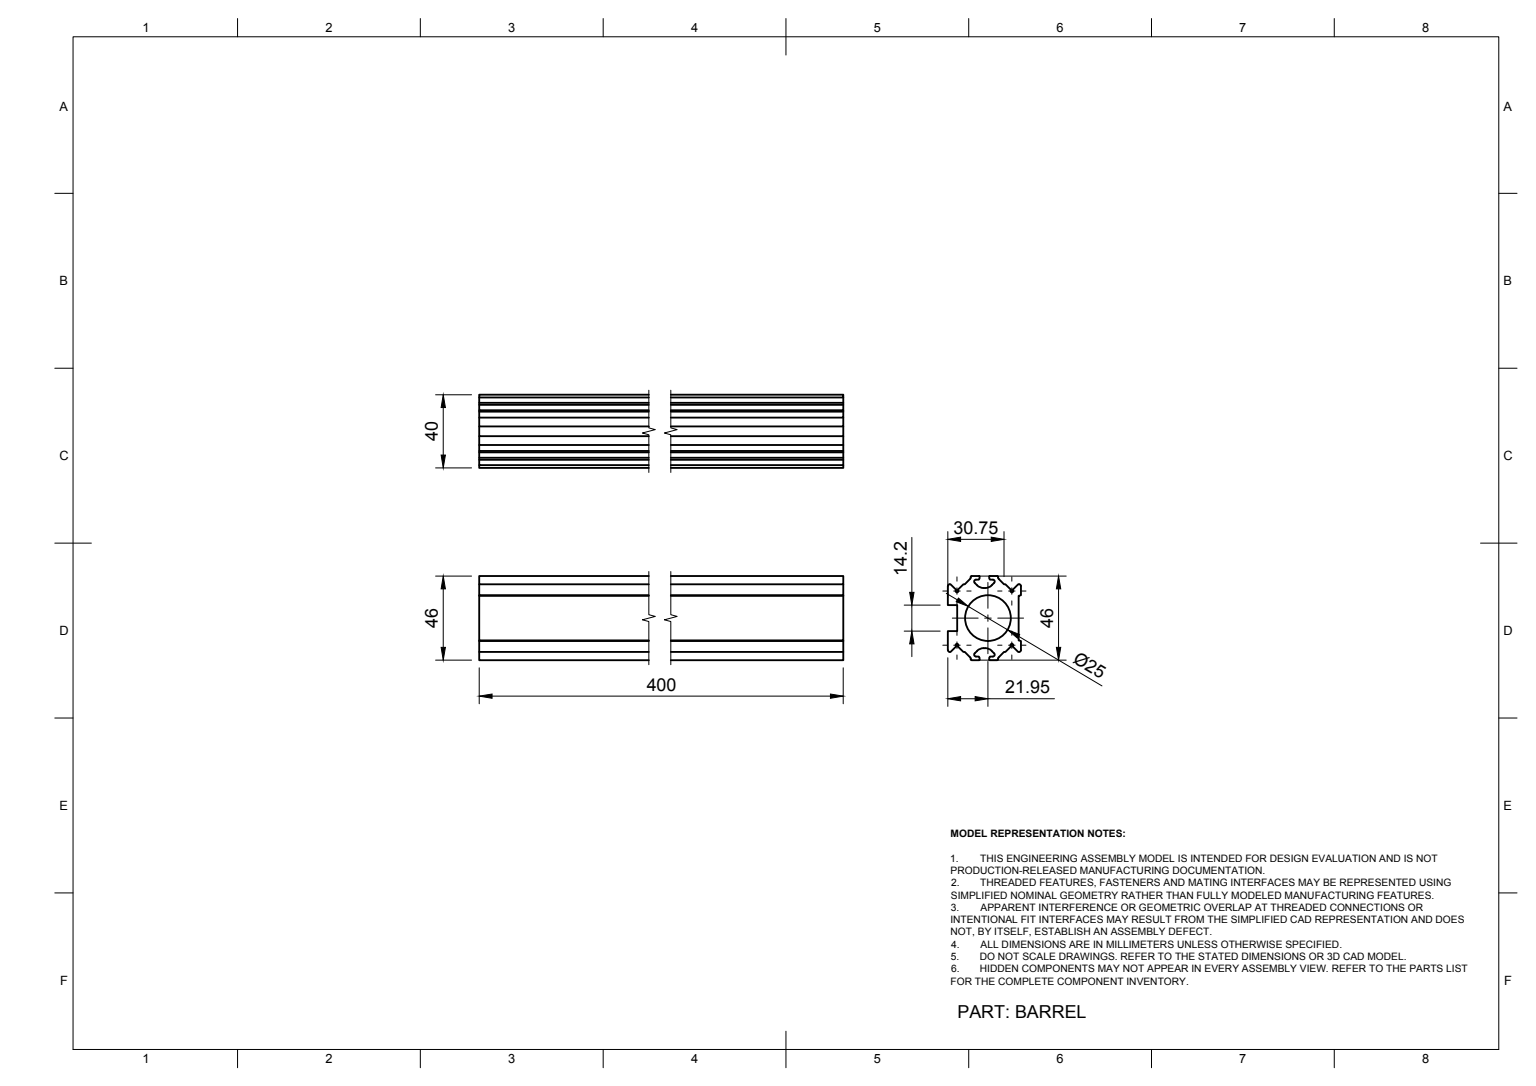
ISO-10303-21;
HEADER;
/* Generated by software containing ST-Developer
 * from STEP Tools, Inc. (www.steptools.com) 
 */

FILE_DESCRIPTION(
/* description */ (''),
/* implementation_level */ '2;1');

FILE_NAME(
/* name */ 'Barrel.step',
/* time_stamp */ '2026-10-05T11:01:41-07:00',
/* author */ (''),
/* organization */ (''),
/* preprocessor_version */ 'ST-DEVELOPER v20.2',
/* originating_system */ 'Autodesk Translation Framework v15.15.0.0',
/* authorisation */ '');

FILE_SCHEMA (('AUTOMOTIVE_DESIGN { 1 0 10303 214 3 1 1 }'));
ENDSEC;

DATA;
#10=MECHANICAL_DESIGN_GEOMETRIC_PRESENTATION_REPRESENTATION('',(#2144),#215609);
#218=FACE_BOUND('',#5274,.T.);
#219=FACE_BOUND('',#5276,.T.);
#2126=SHAPE_REPRESENTATION_RELATIONSHIP('SRR','None',#215651,#2135);
#2135=ADVANCED_BREP_SHAPE_REPRESENTATION('',(#2153),#215607);
#2144=STYLED_ITEM('',(#215698),#2153);
#2153=MANIFOLD_SOLID_BREP('Body1',#28087);
#2652=CYLINDRICAL_SURFACE('',#29551,12.5);
#2653=CYLINDRICAL_SURFACE('',#29554,0.999999999999998);
#2654=CYLINDRICAL_SURFACE('',#29562,1.);
#2655=CYLINDRICAL_SURFACE('',#29567,0.299999999999999);
#2656=CYLINDRICAL_SURFACE('',#29570,0.75);
#2657=CYLINDRICAL_SURFACE('',#29573,0.300000000000001);
#2658=CYLINDRICAL_SURFACE('',#29579,1.);
#2659=CYLINDRICAL_SURFACE('',#29583,0.499999999999999);
#2660=CYLINDRICAL_SURFACE('',#29587,0.299999999999998);
#2661=CYLINDRICAL_SURFACE('',#29593,0.999999999999998);
#2662=CYLINDRICAL_SURFACE('',#29597,5.);
#2663=CYLINDRICAL_SURFACE('',#29601,5.);
#2664=CYLINDRICAL_SURFACE('',#29605,0.999999999999996);
#2665=CYLINDRICAL_SURFACE('',#29611,0.299999999999998);
#2666=CYLINDRICAL_SURFACE('',#29615,0.5);
#2667=CYLINDRICAL_SURFACE('',#29619,1.);
#2668=CYLINDRICAL_SURFACE('',#29625,0.300000000000002);
#2669=CYLINDRICAL_SURFACE('',#29628,0.75000062202425);
#2670=CYLINDRICAL_SURFACE('',#29631,0.300000000000001);
#2671=CYLINDRICAL_SURFACE('',#29636,1.);
#2672=CYLINDRICAL_SURFACE('',#29644,1.);
#2673=CYLINDRICAL_SURFACE('',#29649,0.300000000000002);
#2674=CYLINDRICAL_SURFACE('',#29652,0.75);
#2675=CYLINDRICAL_SURFACE('',#29655,0.300000000000001);
#2676=CYLINDRICAL_SURFACE('',#29661,1.);
#2677=CYLINDRICAL_SURFACE('',#29665,0.500000000000003);
#2678=CYLINDRICAL_SURFACE('',#29669,0.299999999999998);
#2679=CYLINDRICAL_SURFACE('',#29675,1.);
#2680=CYLINDRICAL_SURFACE('',#29679,4.99999999999999);
#2681=CYLINDRICAL_SURFACE('',#29683,4.99999999999999);
#2682=CYLINDRICAL_SURFACE('',#29687,1.);
#2683=CYLINDRICAL_SURFACE('',#29693,0.300000000000003);
#2684=CYLINDRICAL_SURFACE('',#29697,0.5);
#2685=CYLINDRICAL_SURFACE('',#29701,1.);
#2686=CYLINDRICAL_SURFACE('',#29707,0.300000000000001);
#2687=CYLINDRICAL_SURFACE('',#29710,0.750000622024213);
#2688=CYLINDRICAL_SURFACE('',#29713,0.300000000000001);
#3822=FACE_OUTER_BOUND('',#5180,.T.);
#3823=FACE_OUTER_BOUND('',#5181,.T.);
#3824=FACE_OUTER_BOUND('',#5182,.T.);
#3825=FACE_OUTER_BOUND('',#5183,.T.);
#3826=FACE_OUTER_BOUND('',#5184,.T.);
#3827=FACE_OUTER_BOUND('',#5185,.T.);
#3828=FACE_OUTER_BOUND('',#5186,.T.);
#3829=FACE_OUTER_BOUND('',#5187,.T.);
#3830=FACE_OUTER_BOUND('',#5188,.T.);
#3831=FACE_OUTER_BOUND('',#5189,.T.);
#3832=FACE_OUTER_BOUND('',#5190,.T.);
#3833=FACE_OUTER_BOUND('',#5191,.T.);
#3834=FACE_OUTER_BOUND('',#5192,.T.);
#3835=FACE_OUTER_BOUND('',#5193,.T.);
#3836=FACE_OUTER_BOUND('',#5194,.T.);
#3837=FACE_OUTER_BOUND('',#5195,.T.);
#3838=FACE_OUTER_BOUND('',#5196,.T.);
#3839=FACE_OUTER_BOUND('',#5197,.T.);
#3840=FACE_OUTER_BOUND('',#5198,.T.);
#3841=FACE_OUTER_BOUND('',#5199,.T.);
#3842=FACE_OUTER_BOUND('',#5200,.T.);
#3843=FACE_OUTER_BOUND('',#5201,.T.);
#3844=FACE_OUTER_BOUND('',#5202,.T.);
#3845=FACE_OUTER_BOUND('',#5203,.T.);
#3846=FACE_OUTER_BOUND('',#5204,.T.);
#3847=FACE_OUTER_BOUND('',#5205,.T.);
#3848=FACE_OUTER_BOUND('',#5206,.T.);
#3849=FACE_OUTER_BOUND('',#5207,.T.);
#3850=FACE_OUTER_BOUND('',#5208,.T.);
#3851=FACE_OUTER_BOUND('',#5209,.T.);
#3852=FACE_OUTER_BOUND('',#5210,.T.);
#3853=FACE_OUTER_BOUND('',#5211,.T.);
#3854=FACE_OUTER_BOUND('',#5212,.T.);
#3855=FACE_OUTER_BOUND('',#5213,.T.);
#3856=FACE_OUTER_BOUND('',#5214,.T.);
#3857=FACE_OUTER_BOUND('',#5215,.T.);
#3858=FACE_OUTER_BOUND('',#5216,.T.);
#3859=FACE_OUTER_BOUND('',#5217,.T.);
#3860=FACE_OUTER_BOUND('',#5218,.T.);
#3861=FACE_OUTER_BOUND('',#5219,.T.);
#3862=FACE_OUTER_BOUND('',#5220,.T.);
#3863=FACE_OUTER_BOUND('',#5221,.T.);
#3864=FACE_OUTER_BOUND('',#5222,.T.);
#3865=FACE_OUTER_BOUND('',#5223,.T.);
#3866=FACE_OUTER_BOUND('',#5224,.T.);
#3867=FACE_OUTER_BOUND('',#5225,.T.);
#3868=FACE_OUTER_BOUND('',#5226,.T.);
#3869=FACE_OUTER_BOUND('',#5227,.T.);
#3870=FACE_OUTER_BOUND('',#5228,.T.);
#3871=FACE_OUTER_BOUND('',#5229,.T.);
#3872=FACE_OUTER_BOUND('',#5230,.T.);
#3873=FACE_OUTER_BOUND('',#5231,.T.);
#3874=FACE_OUTER_BOUND('',#5232,.T.);
#3875=FACE_OUTER_BOUND('',#5233,.T.);
#3876=FACE_OUTER_BOUND('',#5234,.T.);
#3877=FACE_OUTER_BOUND('',#5235,.T.);
#3878=FACE_OUTER_BOUND('',#5236,.T.);
#3879=FACE_OUTER_BOUND('',#5237,.T.);
#3880=FACE_OUTER_BOUND('',#5238,.T.);
#3881=FACE_OUTER_BOUND('',#5239,.T.);
#3882=FACE_OUTER_BOUND('',#5240,.T.);
#3883=FACE_OUTER_BOUND('',#5241,.T.);
#3884=FACE_OUTER_BOUND('',#5242,.T.);
#3885=FACE_OUTER_BOUND('',#5243,.T.);
#3886=FACE_OUTER_BOUND('',#5244,.T.);
#3887=FACE_OUTER_BOUND('',#5245,.T.);
#3888=FACE_OUTER_BOUND('',#5246,.T.);
#3889=FACE_OUTER_BOUND('',#5247,.T.);
#3890=FACE_OUTER_BOUND('',#5248,.T.);
#3891=FACE_OUTER_BOUND('',#5249,.T.);
#3892=FACE_OUTER_BOUND('',#5250,.T.);
#3893=FACE_OUTER_BOUND('',#5251,.T.);
#3894=FACE_OUTER_BOUND('',#5252,.T.);
#3895=FACE_OUTER_BOUND('',#5253,.T.);
#3896=FACE_OUTER_BOUND('',#5254,.T.);
#3897=FACE_OUTER_BOUND('',#5255,.T.);
#3898=FACE_OUTER_BOUND('',#5256,.T.);
#3899=FACE_OUTER_BOUND('',#5257,.T.);
#3900=FACE_OUTER_BOUND('',#5258,.T.);
#3901=FACE_OUTER_BOUND('',#5259,.T.);
#3902=FACE_OUTER_BOUND('',#5260,.T.);
#3903=FACE_OUTER_BOUND('',#5261,.T.);
#3904=FACE_OUTER_BOUND('',#5262,.T.);
#3905=FACE_OUTER_BOUND('',#5263,.T.);
#3906=FACE_OUTER_BOUND('',#5264,.T.);
#3907=FACE_OUTER_BOUND('',#5265,.T.);
#3908=FACE_OUTER_BOUND('',#5266,.T.);
#3909=FACE_OUTER_BOUND('',#5267,.T.);
#3910=FACE_OUTER_BOUND('',#5268,.T.);
#3911=FACE_OUTER_BOUND('',#5269,.T.);
#3912=FACE_OUTER_BOUND('',#5270,.T.);
#3913=FACE_OUTER_BOUND('',#5271,.T.);
#3914=FACE_OUTER_BOUND('',#5272,.T.);
#3915=FACE_OUTER_BOUND('',#5273,.T.);
#3916=FACE_OUTER_BOUND('',#5275,.T.);
#5180=EDGE_LOOP('',(#22991,#22992,#22993,#22994));
#5181=EDGE_LOOP('',(#22995,#22996,#22997,#22998));
#5182=EDGE_LOOP('',(#22999,#23000,#23001,#23002));
#5183=EDGE_LOOP('',(#23003,#23004,#23005,#23006));
#5184=EDGE_LOOP('',(#23007,#23008,#23009,#23010));
#5185=EDGE_LOOP('',(#23011,#23012,#23013,#23014));
#5186=EDGE_LOOP('',(#23015,#23016,#23017,#23018));
#5187=EDGE_LOOP('',(#23019,#23020,#23021,#23022));
#5188=EDGE_LOOP('',(#23023,#23024,#23025,#23026));
#5189=EDGE_LOOP('',(#23027,#23028,#23029,#23030));
#5190=EDGE_LOOP('',(#23031,#23032,#23033,#23034));
#5191=EDGE_LOOP('',(#23035,#23036,#23037,#23038));
#5192=EDGE_LOOP('',(#23039,#23040,#23041,#23042));
#5193=EDGE_LOOP('',(#23043,#23044,#23045,#23046));
#5194=EDGE_LOOP('',(#23047,#23048,#23049,#23050));
#5195=EDGE_LOOP('',(#23051,#23052,#23053,#23054));
#5196=EDGE_LOOP('',(#23055,#23056,#23057,#23058));
#5197=EDGE_LOOP('',(#23059,#23060,#23061,#23062));
#5198=EDGE_LOOP('',(#23063,#23064,#23065,#23066));
#5199=EDGE_LOOP('',(#23067,#23068,#23069,#23070));
#5200=EDGE_LOOP('',(#23071,#23072,#23073,#23074));
#5201=EDGE_LOOP('',(#23075,#23076,#23077,#23078));
#5202=EDGE_LOOP('',(#23079,#23080,#23081,#23082));
#5203=EDGE_LOOP('',(#23083,#23084,#23085,#23086));
#5204=EDGE_LOOP('',(#23087,#23088,#23089,#23090));
#5205=EDGE_LOOP('',(#23091,#23092,#23093,#23094));
#5206=EDGE_LOOP('',(#23095,#23096,#23097,#23098));
#5207=EDGE_LOOP('',(#23099,#23100,#23101,#23102));
#5208=EDGE_LOOP('',(#23103,#23104,#23105,#23106));
#5209=EDGE_LOOP('',(#23107,#23108,#23109,#23110));
#5210=EDGE_LOOP('',(#23111,#23112,#23113,#23114));
#5211=EDGE_LOOP('',(#23115,#23116,#23117,#23118));
#5212=EDGE_LOOP('',(#23119,#23120,#23121,#23122));
#5213=EDGE_LOOP('',(#23123,#23124,#23125,#23126));
#5214=EDGE_LOOP('',(#23127,#23128,#23129,#23130));
#5215=EDGE_LOOP('',(#23131,#23132,#23133,#23134));
#5216=EDGE_LOOP('',(#23135,#23136,#23137,#23138));
#5217=EDGE_LOOP('',(#23139,#23140,#23141,#23142));
#5218=EDGE_LOOP('',(#23143,#23144,#23145,#23146));
#5219=EDGE_LOOP('',(#23147,#23148,#23149,#23150));
#5220=EDGE_LOOP('',(#23151,#23152,#23153,#23154));
#5221=EDGE_LOOP('',(#23155,#23156,#23157,#23158));
#5222=EDGE_LOOP('',(#23159,#23160,#23161,#23162));
#5223=EDGE_LOOP('',(#23163,#23164,#23165,#23166));
#5224=EDGE_LOOP('',(#23167,#23168,#23169,#23170));
#5225=EDGE_LOOP('',(#23171,#23172,#23173,#23174));
#5226=EDGE_LOOP('',(#23175,#23176,#23177,#23178));
#5227=EDGE_LOOP('',(#23179,#23180,#23181,#23182));
#5228=EDGE_LOOP('',(#23183,#23184,#23185,#23186));
#5229=EDGE_LOOP('',(#23187,#23188,#23189,#23190));
#5230=EDGE_LOOP('',(#23191,#23192,#23193,#23194));
#5231=EDGE_LOOP('',(#23195,#23196,#23197,#23198));
#5232=EDGE_LOOP('',(#23199,#23200,#23201,#23202));
#5233=EDGE_LOOP('',(#23203,#23204,#23205,#23206));
#5234=EDGE_LOOP('',(#23207,#23208,#23209,#23210));
#5235=EDGE_LOOP('',(#23211,#23212,#23213,#23214));
#5236=EDGE_LOOP('',(#23215,#23216,#23217,#23218));
#5237=EDGE_LOOP('',(#23219,#23220,#23221,#23222));
#5238=EDGE_LOOP('',(#23223,#23224,#23225,#23226));
#5239=EDGE_LOOP('',(#23227,#23228,#23229,#23230));
#5240=EDGE_LOOP('',(#23231,#23232,#23233,#23234));
#5241=EDGE_LOOP('',(#23235,#23236,#23237,#23238));
#5242=EDGE_LOOP('',(#23239,#23240,#23241,#23242));
#5243=EDGE_LOOP('',(#23243,#23244,#23245,#23246));
#5244=EDGE_LOOP('',(#23247,#23248,#23249,#23250));
#5245=EDGE_LOOP('',(#23251,#23252,#23253,#23254));
#5246=EDGE_LOOP('',(#23255,#23256,#23257,#23258));
#5247=EDGE_LOOP('',(#23259,#23260,#23261,#23262));
#5248=EDGE_LOOP('',(#23263,#23264,#23265,#23266));
#5249=EDGE_LOOP('',(#23267,#23268,#23269,#23270));
#5250=EDGE_LOOP('',(#23271,#23272,#23273,#23274));
#5251=EDGE_LOOP('',(#23275,#23276,#23277,#23278));
#5252=EDGE_LOOP('',(#23279,#23280,#23281,#23282));
#5253=EDGE_LOOP('',(#23283,#23284,#23285,#23286));
#5254=EDGE_LOOP('',(#23287,#23288,#23289,#23290));
#5255=EDGE_LOOP('',(#23291,#23292,#23293,#23294));
#5256=EDGE_LOOP('',(#23295,#23296,#23297,#23298));
#5257=EDGE_LOOP('',(#23299,#23300,#23301,#23302));
#5258=EDGE_LOOP('',(#23303,#23304,#23305,#23306));
#5259=EDGE_LOOP('',(#23307,#23308,#23309,#23310));
#5260=EDGE_LOOP('',(#23311,#23312,#23313,#23314));
#5261=EDGE_LOOP('',(#23315,#23316,#23317,#23318));
#5262=EDGE_LOOP('',(#23319,#23320,#23321,#23322));
#5263=EDGE_LOOP('',(#23323,#23324,#23325,#23326));
#5264=EDGE_LOOP('',(#23327,#23328,#23329,#23330));
#5265=EDGE_LOOP('',(#23331,#23332,#23333,#23334));
#5266=EDGE_LOOP('',(#23335,#23336,#23337,#23338));
#5267=EDGE_LOOP('',(#23339,#23340,#23341,#23342));
#5268=EDGE_LOOP('',(#23343,#23344,#23345,#23346));
#5269=EDGE_LOOP('',(#23347,#23348,#23349,#23350));
#5270=EDGE_LOOP('',(#23351,#23352,#23353,#23354));
#5271=EDGE_LOOP('',(#23355,#23356,#23357,#23358));
#5272=EDGE_LOOP('',(#23359,#23360,#23361,#23362));
#5273=EDGE_LOOP('',(#23363,#23364,#23365,#23366,#23367,#23368,#23369,#23370,
#23371,#23372,#23373,#23374,#23375,#23376,#23377,#23378,#23379,#23380,#23381,
#23382,#23383,#23384,#23385,#23386,#23387,#23388,#23389,#23390,#23391,#23392,
#23393,#23394,#23395,#23396,#23397,#23398,#23399,#23400,#23401,#23402,#23403,
#23404,#23405,#23406,#23407,#23408,#23409,#23410,#23411,#23412,#23413,#23414,
#23415,#23416,#23417,#23418,#23419,#23420,#23421,#23422,#23423,#23424,#23425,
#23426,#23427,#23428,#23429,#23430,#23431,#23432,#23433,#23434,#23435,#23436,
#23437,#23438,#23439,#23440,#23441,#23442,#23443,#23444,#23445,#23446,#23447,
#23448,#23449,#23450,#23451,#23452,#23453,#23454));
#5274=EDGE_LOOP('',(#23455));
#5275=EDGE_LOOP('',(#23456,#23457,#23458,#23459,#23460,#23461,#23462,#23463,
#23464,#23465,#23466,#23467,#23468,#23469,#23470,#23471,#23472,#23473,#23474,
#23475,#23476,#23477,#23478,#23479,#23480,#23481,#23482,#23483,#23484,#23485,
#23486,#23487,#23488,#23489,#23490,#23491,#23492,#23493,#23494,#23495,#23496,
#23497,#23498,#23499,#23500,#23501,#23502,#23503,#23504,#23505,#23506,#23507,
#23508,#23509,#23510,#23511,#23512,#23513,#23514,#23515,#23516,#23517,#23518,
#23519,#23520,#23521,#23522,#23523,#23524,#23525,#23526,#23527,#23528,#23529,
#23530,#23531,#23532,#23533,#23534,#23535,#23536,#23537,#23538,#23539,#23540,
#23541,#23542,#23543,#23544,#23545,#23546,#23547));
#5276=EDGE_LOOP('',(#23548));
#6134=CIRCLE('',#29552,12.5);
#6135=CIRCLE('',#29553,12.5);
#6136=CIRCLE('',#29555,0.999999999999998);
#6137=CIRCLE('',#29556,0.999999999999998);
#6138=CIRCLE('',#29563,1.);
#6139=CIRCLE('',#29564,1.);
#6140=CIRCLE('',#29568,0.299999999999999);
#6141=CIRCLE('',#29569,0.299999999999999);
#6142=CIRCLE('',#29571,0.75);
#6143=CIRCLE('',#29572,0.75);
#6144=CIRCLE('',#29574,0.300000000000001);
#6145=CIRCLE('',#29575,0.300000000000001);
#6146=CIRCLE('',#29580,1.);
#6147=CIRCLE('',#29581,1.);
#6148=CIRCLE('',#29584,0.499999999999999);
#6149=CIRCLE('',#29585,0.499999999999999);
#6150=CIRCLE('',#29588,0.299999999999998);
#6151=CIRCLE('',#29589,0.299999999999998);
#6152=CIRCLE('',#29594,0.999999999999998);
#6153=CIRCLE('',#29595,0.999999999999998);
#6154=CIRCLE('',#29598,5.);
#6155=CIRCLE('',#29599,5.);
#6156=CIRCLE('',#29602,5.);
#6157=CIRCLE('',#29603,5.);
#6158=CIRCLE('',#29606,0.999999999999996);
#6159=CIRCLE('',#29607,0.999999999999996);
#6160=CIRCLE('',#29612,0.299999999999998);
#6161=CIRCLE('',#29613,0.299999999999998);
#6162=CIRCLE('',#29616,0.5);
#6163=CIRCLE('',#29617,0.5);
#6164=CIRCLE('',#29620,1.);
#6165=CIRCLE('',#29621,1.);
#6166=CIRCLE('',#29626,0.300000000000002);
#6167=CIRCLE('',#29627,0.300000000000002);
#6168=CIRCLE('',#29629,0.75000062202425);
#6169=CIRCLE('',#29630,0.75000062202425);
#6170=CIRCLE('',#29632,0.300000000000001);
#6171=CIRCLE('',#29633,0.300000000000001);
#6172=CIRCLE('',#29637,1.);
#6173=CIRCLE('',#29638,1.);
#6174=CIRCLE('',#29645,1.);
#6175=CIRCLE('',#29646,1.);
#6176=CIRCLE('',#29650,0.300000000000002);
#6177=CIRCLE('',#29651,0.300000000000002);
#6178=CIRCLE('',#29653,0.75);
#6179=CIRCLE('',#29654,0.75);
#6180=CIRCLE('',#29656,0.300000000000001);
#6181=CIRCLE('',#29657,0.300000000000001);
#6182=CIRCLE('',#29662,1.);
#6183=CIRCLE('',#29663,1.);
#6184=CIRCLE('',#29666,0.500000000000003);
#6185=CIRCLE('',#29667,0.500000000000003);
#6186=CIRCLE('',#29670,0.299999999999998);
#6187=CIRCLE('',#29671,0.299999999999998);
#6188=CIRCLE('',#29676,1.);
#6189=CIRCLE('',#29677,1.);
#6190=CIRCLE('',#29680,4.99999999999999);
#6191=CIRCLE('',#29681,4.99999999999999);
#6192=CIRCLE('',#29684,4.99999999999999);
#6193=CIRCLE('',#29685,4.99999999999999);
#6194=CIRCLE('',#29688,1.);
#6195=CIRCLE('',#29689,1.);
#6196=CIRCLE('',#29694,0.300000000000003);
#6197=CIRCLE('',#29695,0.300000000000003);
#6198=CIRCLE('',#29698,0.5);
#6199=CIRCLE('',#29699,0.5);
#6200=CIRCLE('',#29702,1.);
#6201=CIRCLE('',#29703,1.);
#6202=CIRCLE('',#29708,0.300000000000001);
#6203=CIRCLE('',#29709,0.300000000000001);
#6204=CIRCLE('',#29711,0.750000622024213);
#6205=CIRCLE('',#29712,0.750000622024213);
#6206=CIRCLE('',#29714,0.300000000000001);
#6207=CIRCLE('',#29715,0.300000000000001);
#7517=LINE('',#127846,#9362);
#7518=LINE('',#127853,#9363);
#7519=LINE('',#127856,#9364);
#7520=LINE('',#127859,#9365);
#7521=LINE('',#127861,#9366);
#7522=LINE('',#127862,#9367);
#7523=LINE('',#127865,#9368);
#7524=LINE('',#127867,#9369);
#7525=LINE('',#127868,#9370);
#7526=LINE('',#127871,#9371);
#7527=LINE('',#127873,#9372);
#7528=LINE('',#127874,#9373);
#7529=LINE('',#127877,#9374);
#7530=LINE('',#127879,#9375);
#7531=LINE('',#127880,#9376);
#7532=LINE('',#127883,#9377);
#7533=LINE('',#127885,#9378);
#7534=LINE('',#127886,#9379);
#7535=LINE('',#127892,#9380);
#7536=LINE('',#127895,#9381);
#7537=LINE('',#127897,#9382);
#7538=LINE('',#127898,#9383);
#7539=LINE('',#127901,#9384);
#7540=LINE('',#127903,#9385);
#7541=LINE('',#127904,#9386);
#7542=LINE('',#127910,#9387);
#7543=LINE('',#127916,#9388);
#7544=LINE('',#127922,#9389);
#7545=LINE('',#127925,#9390);
#7546=LINE('',#127927,#9391);
#7547=LINE('',#127928,#9392);
#7548=LINE('',#127931,#9393);
#7549=LINE('',#127933,#9394);
#7550=LINE('',#127934,#9395);
#7551=LINE('',#127937,#9396);
#7552=LINE('',#127939,#9397);
#7553=LINE('',#127940,#9398);
#7554=LINE('',#127946,#9399);
#7555=LINE('',#127949,#9400);
#7556=LINE('',#127951,#9401);
#7557=LINE('',#127952,#9402);
#7558=LINE('',#127958,#9403);
#7559=LINE('',#127961,#9404);
#7560=LINE('',#127963,#9405);
#7561=LINE('',#127964,#9406);
#7562=LINE('',#127970,#9407);
#7563=LINE('',#127973,#9408);
#7564=LINE('',#127975,#9409);
#7565=LINE('',#127976,#9410);
#7566=LINE('',#127979,#9411);
#7567=LINE('',#127981,#9412);
#7568=LINE('',#127982,#9413);
#7569=LINE('',#127985,#9414);
#7570=LINE('',#127987,#9415);
#7571=LINE('',#127988,#9416);
#7572=LINE('',#127994,#9417);
#7573=LINE('',#127997,#9418);
#7574=LINE('',#127999,#9419);
#7575=LINE('',#128000,#9420);
#7576=LINE('',#128006,#9421);
#7577=LINE('',#128009,#9422);
#7578=LINE('',#128011,#9423);
#7579=LINE('',#128012,#9424);
#7580=LINE('',#128018,#9425);
#7581=LINE('',#128021,#9426);
#7582=LINE('',#128023,#9427);
#7583=LINE('',#128024,#9428);
#7584=LINE('',#128030,#9429);
#7585=LINE('',#128033,#9430);
#7586=LINE('',#128035,#9431);
#7587=LINE('',#128036,#9432);
#7588=LINE('',#128039,#9433);
#7589=LINE('',#128041,#9434);
#7590=LINE('',#128042,#9435);
#7591=LINE('',#128045,#9436);
#7592=LINE('',#128047,#9437);
#7593=LINE('',#128048,#9438);
#7594=LINE('',#128054,#9439);
#7595=LINE('',#128057,#9440);
#7596=LINE('',#128059,#9441);
#7597=LINE('',#128060,#9442);
#7598=LINE('',#128066,#9443);
#7599=LINE('',#128069,#9444);
#7600=LINE('',#128071,#9445);
#7601=LINE('',#128072,#9446);
#7602=LINE('',#128078,#9447);
#7603=LINE('',#128081,#9448);
#7604=LINE('',#128083,#9449);
#7605=LINE('',#128084,#9450);
#7606=LINE('',#128087,#9451);
#7607=LINE('',#128089,#9452);
#7608=LINE('',#128090,#9453);
#7609=LINE('',#128093,#9454);
#7610=LINE('',#128095,#9455);
#7611=LINE('',#128096,#9456);
#7612=LINE('',#128102,#9457);
#7613=LINE('',#128108,#9458);
#7614=LINE('',#128114,#9459);
#7615=LINE('',#128117,#9460);
#7616=LINE('',#128119,#9461);
#7617=LINE('',#128120,#9462);
#7618=LINE('',#128123,#9463);
#7619=LINE('',#128125,#9464);
#7620=LINE('',#128126,#9465);
#7621=LINE('',#128132,#9466);
#7622=LINE('',#128135,#9467);
#7623=LINE('',#128137,#9468);
#7624=LINE('',#128138,#9469);
#7625=LINE('',#128141,#9470);
#7626=LINE('',#128143,#9471);
#7627=LINE('',#128144,#9472);
#7628=LINE('',#128147,#9473);
#7629=LINE('',#128149,#9474);
#7630=LINE('',#128150,#9475);
#7631=LINE('',#128153,#9476);
#7632=LINE('',#128155,#9477);
#7633=LINE('',#128156,#9478);
#7634=LINE('',#128159,#9479);
#7635=LINE('',#128161,#9480);
#7636=LINE('',#128162,#9481);
#7637=LINE('',#128168,#9482);
#7638=LINE('',#128171,#9483);
#7639=LINE('',#128173,#9484);
#7640=LINE('',#128174,#9485);
#7641=LINE('',#128177,#9486);
#7642=LINE('',#128179,#9487);
#7643=LINE('',#128180,#9488);
#7644=LINE('',#128186,#9489);
#7645=LINE('',#128192,#9490);
#7646=LINE('',#128198,#9491);
#7647=LINE('',#128201,#9492);
#7648=LINE('',#128203,#9493);
#7649=LINE('',#128204,#9494);
#7650=LINE('',#128207,#9495);
#7651=LINE('',#128209,#9496);
#7652=LINE('',#128210,#9497);
#7653=LINE('',#128213,#9498);
#7654=LINE('',#128215,#9499);
#7655=LINE('',#128216,#9500);
#7656=LINE('',#128222,#9501);
#7657=LINE('',#128225,#9502);
#7658=LINE('',#128227,#9503);
#7659=LINE('',#128228,#9504);
#7660=LINE('',#128234,#9505);
#7661=LINE('',#128237,#9506);
#7662=LINE('',#128239,#9507);
#7663=LINE('',#128240,#9508);
#7664=LINE('',#128246,#9509);
#7665=LINE('',#128249,#9510);
#7666=LINE('',#128251,#9511);
#7667=LINE('',#128252,#9512);
#7668=LINE('',#128255,#9513);
#7669=LINE('',#128257,#9514);
#7670=LINE('',#128258,#9515);
#7671=LINE('',#128261,#9516);
#7672=LINE('',#128263,#9517);
#7673=LINE('',#128264,#9518);
#7674=LINE('',#128270,#9519);
#7675=LINE('',#128273,#9520);
#7676=LINE('',#128275,#9521);
#7677=LINE('',#128276,#9522);
#7678=LINE('',#128282,#9523);
#7679=LINE('',#128285,#9524);
#7680=LINE('',#128287,#9525);
#7681=LINE('',#128288,#9526);
#7682=LINE('',#128294,#9527);
#7683=LINE('',#128297,#9528);
#7684=LINE('',#128299,#9529);
#7685=LINE('',#128300,#9530);
#7686=LINE('',#128306,#9531);
#7687=LINE('',#128309,#9532);
#7688=LINE('',#128311,#9533);
#7689=LINE('',#128312,#9534);
#7690=LINE('',#128315,#9535);
#7691=LINE('',#128317,#9536);
#7692=LINE('',#128318,#9537);
#7693=LINE('',#128321,#9538);
#7694=LINE('',#128323,#9539);
#7695=LINE('',#128324,#9540);
#7696=LINE('',#128330,#9541);
#7697=LINE('',#128333,#9542);
#7698=LINE('',#128335,#9543);
#7699=LINE('',#128336,#9544);
#7700=LINE('',#128342,#9545);
#7701=LINE('',#128345,#9546);
#7702=LINE('',#128347,#9547);
#7703=LINE('',#128348,#9548);
#7704=LINE('',#128354,#9549);
#7705=LINE('',#128357,#9550);
#7706=LINE('',#128359,#9551);
#7707=LINE('',#128360,#9552);
#7708=LINE('',#128363,#9553);
#7709=LINE('',#128365,#9554);
#7710=LINE('',#128366,#9555);
#7711=LINE('',#128369,#9556);
#7712=LINE('',#128371,#9557);
#7713=LINE('',#128372,#9558);
#7714=LINE('',#128378,#9559);
#7715=LINE('',#128384,#9560);
#7716=LINE('',#128390,#9561);
#7717=LINE('',#128393,#9562);
#7718=LINE('',#128395,#9563);
#7719=LINE('',#128396,#9564);
#7720=LINE('',#128398,#9565);
#7721=LINE('',#128399,#9566);
#9362=VECTOR('',#34135,12.5);
#9363=VECTOR('',#34142,10.);
#9364=VECTOR('',#34145,10.);
#9365=VECTOR('',#34148,10.);
#9366=VECTOR('',#34149,10.);
#9367=VECTOR('',#34150,10.);
#9368=VECTOR('',#34153,10.);
#9369=VECTOR('',#34154,10.);
#9370=VECTOR('',#34155,10.);
#9371=VECTOR('',#34158,10.);
#9372=VECTOR('',#34159,10.);
#9373=VECTOR('',#34160,10.);
#9374=VECTOR('',#34163,10.);
#9375=VECTOR('',#34164,10.);
#9376=VECTOR('',#34165,10.);
#9377=VECTOR('',#34168,10.);
#9378=VECTOR('',#34169,10.);
#9379=VECTOR('',#34170,10.);
#9380=VECTOR('',#34177,10.);
#9381=VECTOR('',#34180,10.);
#9382=VECTOR('',#34181,10.);
#9383=VECTOR('',#34182,10.);
#9384=VECTOR('',#34185,10.);
#9385=VECTOR('',#34186,10.);
#9386=VECTOR('',#34187,10.);
#9387=VECTOR('',#34194,10.);
#9388=VECTOR('',#34201,10.);
#9389=VECTOR('',#34208,10.);
#9390=VECTOR('',#34211,10.);
#9391=VECTOR('',#34212,10.);
#9392=VECTOR('',#34213,10.);
#9393=VECTOR('',#34216,10.);
#9394=VECTOR('',#34217,10.);
#9395=VECTOR('',#34218,10.);
#9396=VECTOR('',#34221,10.);
#9397=VECTOR('',#34222,10.);
#9398=VECTOR('',#34223,10.);
#9399=VECTOR('',#34230,10.);
#9400=VECTOR('',#34233,10.);
#9401=VECTOR('',#34234,10.);
#9402=VECTOR('',#34235,10.);
#9403=VECTOR('',#34242,10.);
#9404=VECTOR('',#34245,10.);
#9405=VECTOR('',#34246,10.);
#9406=VECTOR('',#34247,10.);
#9407=VECTOR('',#34254,10.);
#9408=VECTOR('',#34257,10.);
#9409=VECTOR('',#34258,10.);
#9410=VECTOR('',#34259,10.);
#9411=VECTOR('',#34262,10.);
#9412=VECTOR('',#34263,10.);
#9413=VECTOR('',#34264,10.);
#9414=VECTOR('',#34267,10.);
#9415=VECTOR('',#34268,10.);
#9416=VECTOR('',#34269,10.);
#9417=VECTOR('',#34276,10.);
#9418=VECTOR('',#34279,10.);
#9419=VECTOR('',#34280,10.);
#9420=VECTOR('',#34281,10.);
#9421=VECTOR('',#34288,10.);
#9422=VECTOR('',#34291,10.);
#9423=VECTOR('',#34292,10.);
#9424=VECTOR('',#34293,10.);
#9425=VECTOR('',#34300,10.);
#9426=VECTOR('',#34303,10.);
#9427=VECTOR('',#34304,10.);
#9428=VECTOR('',#34305,10.);
#9429=VECTOR('',#34312,10.);
#9430=VECTOR('',#34315,10.);
#9431=VECTOR('',#34316,10.);
#9432=VECTOR('',#34317,10.);
#9433=VECTOR('',#34320,10.);
#9434=VECTOR('',#34321,10.);
#9435=VECTOR('',#34322,10.);
#9436=VECTOR('',#34325,10.);
#9437=VECTOR('',#34326,10.);
#9438=VECTOR('',#34327,10.);
#9439=VECTOR('',#34334,10.);
#9440=VECTOR('',#34337,10.);
#9441=VECTOR('',#34338,10.);
#9442=VECTOR('',#34339,10.);
#9443=VECTOR('',#34346,10.);
#9444=VECTOR('',#34349,10.);
#9445=VECTOR('',#34350,10.);
#9446=VECTOR('',#34351,10.);
#9447=VECTOR('',#34358,10.);
#9448=VECTOR('',#34361,10.);
#9449=VECTOR('',#34362,10.);
#9450=VECTOR('',#34363,10.);
#9451=VECTOR('',#34366,10.);
#9452=VECTOR('',#34367,10.);
#9453=VECTOR('',#34368,10.);
#9454=VECTOR('',#34371,9.99999999999999);
#9455=VECTOR('',#34372,9.99999999999999);
#9456=VECTOR('',#34373,10.);
#9457=VECTOR('',#34380,10.);
#9458=VECTOR('',#34387,10.);
#9459=VECTOR('',#34394,10.);
#9460=VECTOR('',#34397,9.99999999999999);
#9461=VECTOR('',#34398,9.99999999999999);
#9462=VECTOR('',#34399,10.);
#9463=VECTOR('',#34402,10.);
#9464=VECTOR('',#34403,10.);
#9465=VECTOR('',#34404,10.);
#9466=VECTOR('',#34411,10.);
#9467=VECTOR('',#34414,10.);
#9468=VECTOR('',#34415,10.);
#9469=VECTOR('',#34416,10.);
#9470=VECTOR('',#34419,10.);
#9471=VECTOR('',#34420,10.);
#9472=VECTOR('',#34421,10.);
#9473=VECTOR('',#34424,10.);
#9474=VECTOR('',#34425,10.);
#9475=VECTOR('',#34426,10.);
#9476=VECTOR('',#34429,10.);
#9477=VECTOR('',#34430,10.);
#9478=VECTOR('',#34431,10.);
#9479=VECTOR('',#34434,10.);
#9480=VECTOR('',#34435,10.);
#9481=VECTOR('',#34436,10.);
#9482=VECTOR('',#34443,10.);
#9483=VECTOR('',#34446,10.);
#9484=VECTOR('',#34447,10.);
#9485=VECTOR('',#34448,10.);
#9486=VECTOR('',#34451,9.99999999999999);
#9487=VECTOR('',#34452,9.99999999999999);
#9488=VECTOR('',#34453,10.);
#9489=VECTOR('',#34460,10.);
#9490=VECTOR('',#34467,10.);
#9491=VECTOR('',#34474,10.);
#9492=VECTOR('',#34477,9.99999999999999);
#9493=VECTOR('',#34478,9.99999999999999);
#9494=VECTOR('',#34479,10.);
#9495=VECTOR('',#34482,10.);
#9496=VECTOR('',#34483,10.);
#9497=VECTOR('',#34484,10.);
#9498=VECTOR('',#34487,10.);
#9499=VECTOR('',#34488,10.);
#9500=VECTOR('',#34489,10.);
#9501=VECTOR('',#34496,10.);
#9502=VECTOR('',#34499,10.);
#9503=VECTOR('',#34500,10.);
#9504=VECTOR('',#34501,10.);
#9505=VECTOR('',#34508,10.);
#9506=VECTOR('',#34511,10.);
#9507=VECTOR('',#34512,10.);
#9508=VECTOR('',#34513,10.);
#9509=VECTOR('',#34520,10.);
#9510=VECTOR('',#34523,10.);
#9511=VECTOR('',#34524,10.);
#9512=VECTOR('',#34525,10.);
#9513=VECTOR('',#34528,10.);
#9514=VECTOR('',#34529,10.);
#9515=VECTOR('',#34530,10.);
#9516=VECTOR('',#34533,10.);
#9517=VECTOR('',#34534,10.);
#9518=VECTOR('',#34535,10.);
#9519=VECTOR('',#34542,10.);
#9520=VECTOR('',#34545,10.);
#9521=VECTOR('',#34546,10.);
#9522=VECTOR('',#34547,10.);
#9523=VECTOR('',#34554,10.);
#9524=VECTOR('',#34557,10.);
#9525=VECTOR('',#34558,10.);
#9526=VECTOR('',#34559,10.);
#9527=VECTOR('',#34566,10.);
#9528=VECTOR('',#34569,10.);
#9529=VECTOR('',#34570,10.);
#9530=VECTOR('',#34571,10.);
#9531=VECTOR('',#34578,10.);
#9532=VECTOR('',#34581,10.);
#9533=VECTOR('',#34582,10.);
#9534=VECTOR('',#34583,10.);
#9535=VECTOR('',#34586,10.);
#9536=VECTOR('',#34587,10.);
#9537=VECTOR('',#34588,10.);
#9538=VECTOR('',#34591,10.);
#9539=VECTOR('',#34592,10.);
#9540=VECTOR('',#34593,10.);
#9541=VECTOR('',#34600,10.);
#9542=VECTOR('',#34603,10.);
#9543=VECTOR('',#34604,10.);
#9544=VECTOR('',#34605,10.);
#9545=VECTOR('',#34612,10.);
#9546=VECTOR('',#34615,10.);
#9547=VECTOR('',#34616,10.);
#9548=VECTOR('',#34617,10.);
#9549=VECTOR('',#34624,10.);
#9550=VECTOR('',#34627,10.);
#9551=VECTOR('',#34628,10.);
#9552=VECTOR('',#34629,10.);
#9553=VECTOR('',#34632,10.);
#9554=VECTOR('',#34633,10.);
#9555=VECTOR('',#34634,10.);
#9556=VECTOR('',#34637,10.);
#9557=VECTOR('',#34638,10.);
#9558=VECTOR('',#34639,10.);
#9559=VECTOR('',#34646,10.);
#9560=VECTOR('',#34653,10.);
#9561=VECTOR('',#34660,10.);
#9562=VECTOR('',#34663,10.);
#9563=VECTOR('',#34664,10.);
#9564=VECTOR('',#34665,10.);
#9565=VECTOR('',#34668,10.);
#9566=VECTOR('',#34669,10.);
#11886=VERTEX_POINT('',#127843);
#11887=VERTEX_POINT('',#127845);
#11888=VERTEX_POINT('',#127849);
#11889=VERTEX_POINT('',#127850);
#11890=VERTEX_POINT('',#127852);
#11891=VERTEX_POINT('',#127854);
#11892=VERTEX_POINT('',#127858);
#11893=VERTEX_POINT('',#127860);
#11894=VERTEX_POINT('',#127864);
#11895=VERTEX_POINT('',#127866);
#11896=VERTEX_POINT('',#127870);
#11897=VERTEX_POINT('',#127872);
#11898=VERTEX_POINT('',#127876);
#11899=VERTEX_POINT('',#127878);
#11900=VERTEX_POINT('',#127882);
#11901=VERTEX_POINT('',#127884);
#11902=VERTEX_POINT('',#127888);
#11903=VERTEX_POINT('',#127890);
#11904=VERTEX_POINT('',#127894);
#11905=VERTEX_POINT('',#127896);
#11906=VERTEX_POINT('',#127900);
#11907=VERTEX_POINT('',#127902);
#11908=VERTEX_POINT('',#127906);
#11909=VERTEX_POINT('',#127908);
#11910=VERTEX_POINT('',#127912);
#11911=VERTEX_POINT('',#127914);
#11912=VERTEX_POINT('',#127918);
#11913=VERTEX_POINT('',#127920);
#11914=VERTEX_POINT('',#127924);
#11915=VERTEX_POINT('',#127926);
#11916=VERTEX_POINT('',#127930);
#11917=VERTEX_POINT('',#127932);
#11918=VERTEX_POINT('',#127936);
#11919=VERTEX_POINT('',#127938);
#11920=VERTEX_POINT('',#127942);
#11921=VERTEX_POINT('',#127944);
#11922=VERTEX_POINT('',#127948);
#11923=VERTEX_POINT('',#127950);
#11924=VERTEX_POINT('',#127954);
#11925=VERTEX_POINT('',#127956);
#11926=VERTEX_POINT('',#127960);
#11927=VERTEX_POINT('',#127962);
#11928=VERTEX_POINT('',#127966);
#11929=VERTEX_POINT('',#127968);
#11930=VERTEX_POINT('',#127972);
#11931=VERTEX_POINT('',#127974);
#11932=VERTEX_POINT('',#127978);
#11933=VERTEX_POINT('',#127980);
#11934=VERTEX_POINT('',#127984);
#11935=VERTEX_POINT('',#127986);
#11936=VERTEX_POINT('',#127990);
#11937=VERTEX_POINT('',#127992);
#11938=VERTEX_POINT('',#127996);
#11939=VERTEX_POINT('',#127998);
#11940=VERTEX_POINT('',#128002);
#11941=VERTEX_POINT('',#128004);
#11942=VERTEX_POINT('',#128008);
#11943=VERTEX_POINT('',#128010);
#11944=VERTEX_POINT('',#128014);
#11945=VERTEX_POINT('',#128016);
#11946=VERTEX_POINT('',#128020);
#11947=VERTEX_POINT('',#128022);
#11948=VERTEX_POINT('',#128026);
#11949=VERTEX_POINT('',#128028);
#11950=VERTEX_POINT('',#128032);
#11951=VERTEX_POINT('',#128034);
#11952=VERTEX_POINT('',#128038);
#11953=VERTEX_POINT('',#128040);
#11954=VERTEX_POINT('',#128044);
#11955=VERTEX_POINT('',#128046);
#11956=VERTEX_POINT('',#128050);
#11957=VERTEX_POINT('',#128052);
#11958=VERTEX_POINT('',#128056);
#11959=VERTEX_POINT('',#128058);
#11960=VERTEX_POINT('',#128062);
#11961=VERTEX_POINT('',#128064);
#11962=VERTEX_POINT('',#128068);
#11963=VERTEX_POINT('',#128070);
#11964=VERTEX_POINT('',#128074);
#11965=VERTEX_POINT('',#128076);
#11966=VERTEX_POINT('',#128080);
#11967=VERTEX_POINT('',#128082);
#11968=VERTEX_POINT('',#128086);
#11969=VERTEX_POINT('',#128088);
#11970=VERTEX_POINT('',#128092);
#11971=VERTEX_POINT('',#128094);
#11972=VERTEX_POINT('',#128098);
#11973=VERTEX_POINT('',#128100);
#11974=VERTEX_POINT('',#128104);
#11975=VERTEX_POINT('',#128106);
#11976=VERTEX_POINT('',#128110);
#11977=VERTEX_POINT('',#128112);
#11978=VERTEX_POINT('',#128116);
#11979=VERTEX_POINT('',#128118);
#11980=VERTEX_POINT('',#128122);
#11981=VERTEX_POINT('',#128124);
#11982=VERTEX_POINT('',#128128);
#11983=VERTEX_POINT('',#128130);
#11984=VERTEX_POINT('',#128134);
#11985=VERTEX_POINT('',#128136);
#11986=VERTEX_POINT('',#128140);
#11987=VERTEX_POINT('',#128142);
#11988=VERTEX_POINT('',#128146);
#11989=VERTEX_POINT('',#128148);
#11990=VERTEX_POINT('',#128152);
#11991=VERTEX_POINT('',#128154);
#11992=VERTEX_POINT('',#128158);
#11993=VERTEX_POINT('',#128160);
#11994=VERTEX_POINT('',#128164);
#11995=VERTEX_POINT('',#128166);
#11996=VERTEX_POINT('',#128170);
#11997=VERTEX_POINT('',#128172);
#11998=VERTEX_POINT('',#128176);
#11999=VERTEX_POINT('',#128178);
#12000=VERTEX_POINT('',#128182);
#12001=VERTEX_POINT('',#128184);
#12002=VERTEX_POINT('',#128188);
#12003=VERTEX_POINT('',#128190);
#12004=VERTEX_POINT('',#128194);
#12005=VERTEX_POINT('',#128196);
#12006=VERTEX_POINT('',#128200);
#12007=VERTEX_POINT('',#128202);
#12008=VERTEX_POINT('',#128206);
#12009=VERTEX_POINT('',#128208);
#12010=VERTEX_POINT('',#128212);
#12011=VERTEX_POINT('',#128214);
#12012=VERTEX_POINT('',#128218);
#12013=VERTEX_POINT('',#128220);
#12014=VERTEX_POINT('',#128224);
#12015=VERTEX_POINT('',#128226);
#12016=VERTEX_POINT('',#128230);
#12017=VERTEX_POINT('',#128232);
#12018=VERTEX_POINT('',#128236);
#12019=VERTEX_POINT('',#128238);
#12020=VERTEX_POINT('',#128242);
#12021=VERTEX_POINT('',#128244);
#12022=VERTEX_POINT('',#128248);
#12023=VERTEX_POINT('',#128250);
#12024=VERTEX_POINT('',#128254);
#12025=VERTEX_POINT('',#128256);
#12026=VERTEX_POINT('',#128260);
#12027=VERTEX_POINT('',#128262);
#12028=VERTEX_POINT('',#128266);
#12029=VERTEX_POINT('',#128268);
#12030=VERTEX_POINT('',#128272);
#12031=VERTEX_POINT('',#128274);
#12032=VERTEX_POINT('',#128278);
#12033=VERTEX_POINT('',#128280);
#12034=VERTEX_POINT('',#128284);
#12035=VERTEX_POINT('',#128286);
#12036=VERTEX_POINT('',#128290);
#12037=VERTEX_POINT('',#128292);
#12038=VERTEX_POINT('',#128296);
#12039=VERTEX_POINT('',#128298);
#12040=VERTEX_POINT('',#128302);
#12041=VERTEX_POINT('',#128304);
#12042=VERTEX_POINT('',#128308);
#12043=VERTEX_POINT('',#128310);
#12044=VERTEX_POINT('',#128314);
#12045=VERTEX_POINT('',#128316);
#12046=VERTEX_POINT('',#128320);
#12047=VERTEX_POINT('',#128322);
#12048=VERTEX_POINT('',#128326);
#12049=VERTEX_POINT('',#128328);
#12050=VERTEX_POINT('',#128332);
#12051=VERTEX_POINT('',#128334);
#12052=VERTEX_POINT('',#128338);
#12053=VERTEX_POINT('',#128340);
#12054=VERTEX_POINT('',#128344);
#12055=VERTEX_POINT('',#128346);
#12056=VERTEX_POINT('',#128350);
#12057=VERTEX_POINT('',#128352);
#12058=VERTEX_POINT('',#128356);
#12059=VERTEX_POINT('',#128358);
#12060=VERTEX_POINT('',#128362);
#12061=VERTEX_POINT('',#128364);
#12062=VERTEX_POINT('',#128368);
#12063=VERTEX_POINT('',#128370);
#12064=VERTEX_POINT('',#128374);
#12065=VERTEX_POINT('',#128376);
#12066=VERTEX_POINT('',#128380);
#12067=VERTEX_POINT('',#128382);
#12068=VERTEX_POINT('',#128386);
#12069=VERTEX_POINT('',#128388);
#12070=VERTEX_POINT('',#128392);
#12071=VERTEX_POINT('',#128394);
#15857=EDGE_CURVE('',#11886,#11886,#6134,.T.);
#15858=EDGE_CURVE('',#11886,#11887,#7517,.T.);
#15859=EDGE_CURVE('',#11887,#11887,#6135,.T.);
#15860=EDGE_CURVE('',#11888,#11889,#6136,.T.);
#15861=EDGE_CURVE('',#11889,#11890,#7518,.T.);
#15862=EDGE_CURVE('',#11891,#11890,#6137,.T.);
#15863=EDGE_CURVE('',#11888,#11891,#7519,.T.);
#15864=EDGE_CURVE('',#11888,#11892,#7520,.T.);
#15865=EDGE_CURVE('',#11893,#11891,#7521,.T.);
#15866=EDGE_CURVE('',#11892,#11893,#7522,.T.);
#15867=EDGE_CURVE('',#11894,#11892,#7523,.T.);
#15868=EDGE_CURVE('',#11895,#11893,#7524,.T.);
#15869=EDGE_CURVE('',#11894,#11895,#7525,.T.);
#15870=EDGE_CURVE('',#11896,#11894,#7526,.T.);
#15871=EDGE_CURVE('',#11897,#11895,#7527,.T.);
#15872=EDGE_CURVE('',#11896,#11897,#7528,.T.);
#15873=EDGE_CURVE('',#11896,#11898,#7529,.T.);
#15874=EDGE_CURVE('',#11899,#11897,#7530,.T.);
#15875=EDGE_CURVE('',#11898,#11899,#7531,.T.);
#15876=EDGE_CURVE('',#11900,#11898,#7532,.T.);
#15877=EDGE_CURVE('',#11901,#11899,#7533,.T.);
#15878=EDGE_CURVE('',#11900,#11901,#7534,.T.);
#15879=EDGE_CURVE('',#11902,#11900,#6138,.T.);
#15880=EDGE_CURVE('',#11903,#11901,#6139,.T.);
#15881=EDGE_CURVE('',#11902,#11903,#7535,.T.);
#15882=EDGE_CURVE('',#11902,#11904,#7536,.T.);
#15883=EDGE_CURVE('',#11905,#11903,#7537,.T.);
#15884=EDGE_CURVE('',#11904,#11905,#7538,.T.);
#15885=EDGE_CURVE('',#11904,#11906,#7539,.T.);
#15886=EDGE_CURVE('',#11907,#11905,#7540,.T.);
#15887=EDGE_CURVE('',#11906,#11907,#7541,.T.);
#15888=EDGE_CURVE('',#11908,#11906,#6140,.T.);
#15889=EDGE_CURVE('',#11909,#11907,#6141,.T.);
#15890=EDGE_CURVE('',#11908,#11909,#7542,.T.);
#15891=EDGE_CURVE('',#11908,#11910,#6142,.T.);
#15892=EDGE_CURVE('',#11911,#11909,#6143,.T.);
#15893=EDGE_CURVE('',#11910,#11911,#7543,.T.);
#15894=EDGE_CURVE('',#11912,#11910,#6144,.T.);
#15895=EDGE_CURVE('',#11913,#11911,#6145,.T.);
#15896=EDGE_CURVE('',#11912,#11913,#7544,.T.);
#15897=EDGE_CURVE('',#11914,#11912,#7545,.T.);
#15898=EDGE_CURVE('',#11915,#11913,#7546,.T.);
#15899=EDGE_CURVE('',#11914,#11915,#7547,.T.);
#15900=EDGE_CURVE('',#11914,#11916,#7548,.T.);
#15901=EDGE_CURVE('',#11917,#11915,#7549,.T.);
#15902=EDGE_CURVE('',#11916,#11917,#7550,.T.);
#15903=EDGE_CURVE('',#11916,#11918,#7551,.T.);
#15904=EDGE_CURVE('',#11919,#11917,#7552,.T.);
#15905=EDGE_CURVE('',#11918,#11919,#7553,.T.);
#15906=EDGE_CURVE('',#11918,#11920,#6146,.T.);
#15907=EDGE_CURVE('',#11921,#11919,#6147,.T.);
#15908=EDGE_CURVE('',#11920,#11921,#7554,.T.);
#15909=EDGE_CURVE('',#11920,#11922,#7555,.T.);
#15910=EDGE_CURVE('',#11923,#11921,#7556,.T.);
#15911=EDGE_CURVE('',#11922,#11923,#7557,.T.);
#15912=EDGE_CURVE('',#11924,#11922,#6148,.T.);
#15913=EDGE_CURVE('',#11925,#11923,#6149,.T.);
#15914=EDGE_CURVE('',#11924,#11925,#7558,.T.);
#15915=EDGE_CURVE('',#11924,#11926,#7559,.T.);
#15916=EDGE_CURVE('',#11927,#11925,#7560,.T.);
#15917=EDGE_CURVE('',#11926,#11927,#7561,.T.);
#15918=EDGE_CURVE('',#11928,#11926,#6150,.T.);
#15919=EDGE_CURVE('',#11929,#11927,#6151,.T.);
#15920=EDGE_CURVE('',#11928,#11929,#7562,.T.);
#15921=EDGE_CURVE('',#11928,#11930,#7563,.T.);
#15922=EDGE_CURVE('',#11931,#11929,#7564,.T.);
#15923=EDGE_CURVE('',#11930,#11931,#7565,.T.);
#15924=EDGE_CURVE('',#11930,#11932,#7566,.T.);
#15925=EDGE_CURVE('',#11933,#11931,#7567,.T.);
#15926=EDGE_CURVE('',#11932,#11933,#7568,.T.);
#15927=EDGE_CURVE('',#11932,#11934,#7569,.T.);
#15928=EDGE_CURVE('',#11935,#11933,#7570,.T.);
#15929=EDGE_CURVE('',#11934,#11935,#7571,.T.);
#15930=EDGE_CURVE('',#11934,#11936,#6152,.T.);
#15931=EDGE_CURVE('',#11937,#11935,#6153,.T.);
#15932=EDGE_CURVE('',#11936,#11937,#7572,.T.);
#15933=EDGE_CURVE('',#11936,#11938,#7573,.T.);
#15934=EDGE_CURVE('',#11939,#11937,#7574,.T.);
#15935=EDGE_CURVE('',#11938,#11939,#7575,.T.);
#15936=EDGE_CURVE('',#11938,#11940,#6154,.T.);
#15937=EDGE_CURVE('',#11941,#11939,#6155,.T.);
#15938=EDGE_CURVE('',#11940,#11941,#7576,.T.);
#15939=EDGE_CURVE('',#11942,#11940,#7577,.T.);
#15940=EDGE_CURVE('',#11943,#11941,#7578,.T.);
#15941=EDGE_CURVE('',#11942,#11943,#7579,.T.);
#15942=EDGE_CURVE('',#11942,#11944,#6156,.T.);
#15943=EDGE_CURVE('',#11945,#11943,#6157,.T.);
#15944=EDGE_CURVE('',#11944,#11945,#7580,.T.);
#15945=EDGE_CURVE('',#11946,#11944,#7581,.T.);
#15946=EDGE_CURVE('',#11947,#11945,#7582,.T.);
#15947=EDGE_CURVE('',#11946,#11947,#7583,.T.);
#15948=EDGE_CURVE('',#11946,#11948,#6158,.T.);
#15949=EDGE_CURVE('',#11949,#11947,#6159,.T.);
#15950=EDGE_CURVE('',#11948,#11949,#7584,.T.);
#15951=EDGE_CURVE('',#11950,#11948,#7585,.T.);
#15952=EDGE_CURVE('',#11951,#11949,#7586,.T.);
#15953=EDGE_CURVE('',#11950,#11951,#7587,.T.);
#15954=EDGE_CURVE('',#11952,#11950,#7588,.T.);
#15955=EDGE_CURVE('',#11953,#11951,#7589,.T.);
#15956=EDGE_CURVE('',#11952,#11953,#7590,.T.);
#15957=EDGE_CURVE('',#11954,#11952,#7591,.T.);
#15958=EDGE_CURVE('',#11955,#11953,#7592,.T.);
#15959=EDGE_CURVE('',#11954,#11955,#7593,.T.);
#15960=EDGE_CURVE('',#11956,#11954,#6160,.T.);
#15961=EDGE_CURVE('',#11957,#11955,#6161,.T.);
#15962=EDGE_CURVE('',#11956,#11957,#7594,.T.);
#15963=EDGE_CURVE('',#11958,#11956,#7595,.T.);
#15964=EDGE_CURVE('',#11959,#11957,#7596,.T.);
#15965=EDGE_CURVE('',#11958,#11959,#7597,.T.);
#15966=EDGE_CURVE('',#11960,#11958,#6162,.T.);
#15967=EDGE_CURVE('',#11961,#11959,#6163,.T.);
#15968=EDGE_CURVE('',#11960,#11961,#7598,.T.);
#15969=EDGE_CURVE('',#11962,#11960,#7599,.T.);
#15970=EDGE_CURVE('',#11963,#11961,#7600,.T.);
#15971=EDGE_CURVE('',#11962,#11963,#7601,.T.);
#15972=EDGE_CURVE('',#11962,#11964,#6164,.T.);
#15973=EDGE_CURVE('',#11965,#11963,#6165,.T.);
#15974=EDGE_CURVE('',#11964,#11965,#7602,.T.);
#15975=EDGE_CURVE('',#11966,#11964,#7603,.T.);
#15976=EDGE_CURVE('',#11967,#11965,#7604,.T.);
#15977=EDGE_CURVE('',#11966,#11967,#7605,.T.);
#15978=EDGE_CURVE('',#11968,#11966,#7606,.T.);
#15979=EDGE_CURVE('',#11969,#11967,#7607,.T.);
#15980=EDGE_CURVE('',#11968,#11969,#7608,.T.);
#15981=EDGE_CURVE('',#11968,#11970,#7609,.T.);
#15982=EDGE_CURVE('',#11971,#11969,#7610,.T.);
#15983=EDGE_CURVE('',#11970,#11971,#7611,.T.);
#15984=EDGE_CURVE('',#11972,#11970,#6166,.T.);
#15985=EDGE_CURVE('',#11973,#11971,#6167,.T.);
#15986=EDGE_CURVE('',#11972,#11973,#7612,.T.);
#15987=EDGE_CURVE('',#11972,#11974,#6168,.T.);
#15988=EDGE_CURVE('',#11975,#11973,#6169,.T.);
#15989=EDGE_CURVE('',#11974,#11975,#7613,.T.);
#15990=EDGE_CURVE('',#11976,#11974,#6170,.T.);
#15991=EDGE_CURVE('',#11977,#11975,#6171,.T.);
#15992=EDGE_CURVE('',#11976,#11977,#7614,.T.);
#15993=EDGE_CURVE('',#11978,#11976,#7615,.T.);
#15994=EDGE_CURVE('',#11979,#11977,#7616,.T.);
#15995=EDGE_CURVE('',#11978,#11979,#7617,.T.);
#15996=EDGE_CURVE('',#11980,#11978,#7618,.T.);
#15997=EDGE_CURVE('',#11981,#11979,#7619,.T.);
#15998=EDGE_CURVE('',#11980,#11981,#7620,.T.);
#15999=EDGE_CURVE('',#11982,#11980,#6172,.T.);
#16000=EDGE_CURVE('',#11983,#11981,#6173,.T.);
#16001=EDGE_CURVE('',#11982,#11983,#7621,.T.);
#16002=EDGE_CURVE('',#11984,#11982,#7622,.T.);
#16003=EDGE_CURVE('',#11985,#11983,#7623,.T.);
#16004=EDGE_CURVE('',#11984,#11985,#7624,.T.);
#16005=EDGE_CURVE('',#11986,#11984,#7625,.T.);
#16006=EDGE_CURVE('',#11987,#11985,#7626,.T.);
#16007=EDGE_CURVE('',#11986,#11987,#7627,.T.);
#16008=EDGE_CURVE('',#11986,#11988,#7628,.T.);
#16009=EDGE_CURVE('',#11989,#11987,#7629,.T.);
#16010=EDGE_CURVE('',#11988,#11989,#7630,.T.);
#16011=EDGE_CURVE('',#11988,#11990,#7631,.T.);
#16012=EDGE_CURVE('',#11991,#11989,#7632,.T.);
#16013=EDGE_CURVE('',#11990,#11991,#7633,.T.);
#16014=EDGE_CURVE('',#11990,#11992,#7634,.T.);
#16015=EDGE_CURVE('',#11993,#11991,#7635,.T.);
#16016=EDGE_CURVE('',#11992,#11993,#7636,.T.);
#16017=EDGE_CURVE('',#11994,#11992,#6174,.T.);
#16018=EDGE_CURVE('',#11995,#11993,#6175,.T.);
#16019=EDGE_CURVE('',#11994,#11995,#7637,.T.);
#16020=EDGE_CURVE('',#11994,#11996,#7638,.T.);
#16021=EDGE_CURVE('',#11997,#11995,#7639,.T.);
#16022=EDGE_CURVE('',#11996,#11997,#7640,.T.);
#16023=EDGE_CURVE('',#11996,#11998,#7641,.T.);
#16024=EDGE_CURVE('',#11999,#11997,#7642,.T.);
#16025=EDGE_CURVE('',#11998,#11999,#7643,.T.);
#16026=EDGE_CURVE('',#12000,#11998,#6176,.T.);
#16027=EDGE_CURVE('',#12001,#11999,#6177,.T.);
#16028=EDGE_CURVE('',#12000,#12001,#7644,.T.);
#16029=EDGE_CURVE('',#12000,#12002,#6178,.T.);
#16030=EDGE_CURVE('',#12003,#12001,#6179,.T.);
#16031=EDGE_CURVE('',#12002,#12003,#7645,.T.);
#16032=EDGE_CURVE('',#12004,#12002,#6180,.T.);
#16033=EDGE_CURVE('',#12005,#12003,#6181,.T.);
#16034=EDGE_CURVE('',#12004,#12005,#7646,.T.);
#16035=EDGE_CURVE('',#12006,#12004,#7647,.T.);
#16036=EDGE_CURVE('',#12007,#12005,#7648,.T.);
#16037=EDGE_CURVE('',#12006,#12007,#7649,.T.);
#16038=EDGE_CURVE('',#12006,#12008,#7650,.T.);
#16039=EDGE_CURVE('',#12009,#12007,#7651,.T.);
#16040=EDGE_CURVE('',#12008,#12009,#7652,.T.);
#16041=EDGE_CURVE('',#12008,#12010,#7653,.T.);
#16042=EDGE_CURVE('',#12011,#12009,#7654,.T.);
#16043=EDGE_CURVE('',#12010,#12011,#7655,.T.);
#16044=EDGE_CURVE('',#12010,#12012,#6182,.T.);
#16045=EDGE_CURVE('',#12013,#12011,#6183,.T.);
#16046=EDGE_CURVE('',#12012,#12013,#7656,.T.);
#16047=EDGE_CURVE('',#12012,#12014,#7657,.T.);
#16048=EDGE_CURVE('',#12015,#12013,#7658,.T.);
#16049=EDGE_CURVE('',#12014,#12015,#7659,.T.);
#16050=EDGE_CURVE('',#12016,#12014,#6184,.T.);
#16051=EDGE_CURVE('',#12017,#12015,#6185,.T.);
#16052=EDGE_CURVE('',#12016,#12017,#7660,.T.);
#16053=EDGE_CURVE('',#12016,#12018,#7661,.T.);
#16054=EDGE_CURVE('',#12019,#12017,#7662,.T.);
#16055=EDGE_CURVE('',#12018,#12019,#7663,.T.);
#16056=EDGE_CURVE('',#12020,#12018,#6186,.T.);
#16057=EDGE_CURVE('',#12021,#12019,#6187,.T.);
#16058=EDGE_CURVE('',#12020,#12021,#7664,.T.);
#16059=EDGE_CURVE('',#12020,#12022,#7665,.T.);
#16060=EDGE_CURVE('',#12023,#12021,#7666,.T.);
#16061=EDGE_CURVE('',#12022,#12023,#7667,.T.);
#16062=EDGE_CURVE('',#12022,#12024,#7668,.T.);
#16063=EDGE_CURVE('',#12025,#12023,#7669,.T.);
#16064=EDGE_CURVE('',#12024,#12025,#7670,.T.);
#16065=EDGE_CURVE('',#12024,#12026,#7671,.T.);
#16066=EDGE_CURVE('',#12027,#12025,#7672,.T.);
#16067=EDGE_CURVE('',#12026,#12027,#7673,.T.);
#16068=EDGE_CURVE('',#12026,#12028,#6188,.T.);
#16069=EDGE_CURVE('',#12029,#12027,#6189,.T.);
#16070=EDGE_CURVE('',#12028,#12029,#7674,.T.);
#16071=EDGE_CURVE('',#12028,#12030,#7675,.T.);
#16072=EDGE_CURVE('',#12031,#12029,#7676,.T.);
#16073=EDGE_CURVE('',#12030,#12031,#7677,.T.);
#16074=EDGE_CURVE('',#12030,#12032,#6190,.T.);
#16075=EDGE_CURVE('',#12033,#12031,#6191,.T.);
#16076=EDGE_CURVE('',#12032,#12033,#7678,.T.);
#16077=EDGE_CURVE('',#12032,#12034,#7679,.T.);
#16078=EDGE_CURVE('',#12035,#12033,#7680,.T.);
#16079=EDGE_CURVE('',#12034,#12035,#7681,.T.);
#16080=EDGE_CURVE('',#12034,#12036,#6192,.T.);
#16081=EDGE_CURVE('',#12037,#12035,#6193,.T.);
#16082=EDGE_CURVE('',#12036,#12037,#7682,.T.);
#16083=EDGE_CURVE('',#12038,#12036,#7683,.T.);
#16084=EDGE_CURVE('',#12039,#12037,#7684,.T.);
#16085=EDGE_CURVE('',#12038,#12039,#7685,.T.);
#16086=EDGE_CURVE('',#12038,#12040,#6194,.T.);
#16087=EDGE_CURVE('',#12041,#12039,#6195,.T.);
#16088=EDGE_CURVE('',#12040,#12041,#7686,.T.);
#16089=EDGE_CURVE('',#12042,#12040,#7687,.T.);
#16090=EDGE_CURVE('',#12043,#12041,#7688,.T.);
#16091=EDGE_CURVE('',#12042,#12043,#7689,.T.);
#16092=EDGE_CURVE('',#12044,#12042,#7690,.T.);
#16093=EDGE_CURVE('',#12045,#12043,#7691,.T.);
#16094=EDGE_CURVE('',#12044,#12045,#7692,.T.);
#16095=EDGE_CURVE('',#12046,#12044,#7693,.T.);
#16096=EDGE_CURVE('',#12047,#12045,#7694,.T.);
#16097=EDGE_CURVE('',#12046,#12047,#7695,.T.);
#16098=EDGE_CURVE('',#12048,#12046,#6196,.T.);
#16099=EDGE_CURVE('',#12049,#12047,#6197,.T.);
#16100=EDGE_CURVE('',#12048,#12049,#7696,.T.);
#16101=EDGE_CURVE('',#12050,#12048,#7697,.T.);
#16102=EDGE_CURVE('',#12051,#12049,#7698,.T.);
#16103=EDGE_CURVE('',#12050,#12051,#7699,.T.);
#16104=EDGE_CURVE('',#12052,#12050,#6198,.T.);
#16105=EDGE_CURVE('',#12053,#12051,#6199,.T.);
#16106=EDGE_CURVE('',#12052,#12053,#7700,.T.);
#16107=EDGE_CURVE('',#12054,#12052,#7701,.T.);
#16108=EDGE_CURVE('',#12055,#12053,#7702,.T.);
#16109=EDGE_CURVE('',#12054,#12055,#7703,.T.);
#16110=EDGE_CURVE('',#12054,#12056,#6200,.T.);
#16111=EDGE_CURVE('',#12057,#12055,#6201,.T.);
#16112=EDGE_CURVE('',#12056,#12057,#7704,.T.);
#16113=EDGE_CURVE('',#12058,#12056,#7705,.T.);
#16114=EDGE_CURVE('',#12059,#12057,#7706,.T.);
#16115=EDGE_CURVE('',#12058,#12059,#7707,.T.);
#16116=EDGE_CURVE('',#12060,#12058,#7708,.T.);
#16117=EDGE_CURVE('',#12061,#12059,#7709,.T.);
#16118=EDGE_CURVE('',#12060,#12061,#7710,.T.);
#16119=EDGE_CURVE('',#12060,#12062,#7711,.T.);
#16120=EDGE_CURVE('',#12063,#12061,#7712,.T.);
#16121=EDGE_CURVE('',#12062,#12063,#7713,.T.);
#16122=EDGE_CURVE('',#12064,#12062,#6202,.T.);
#16123=EDGE_CURVE('',#12065,#12063,#6203,.T.);
#16124=EDGE_CURVE('',#12064,#12065,#7714,.T.);
#16125=EDGE_CURVE('',#12064,#12066,#6204,.T.);
#16126=EDGE_CURVE('',#12067,#12065,#6205,.T.);
#16127=EDGE_CURVE('',#12066,#12067,#7715,.T.);
#16128=EDGE_CURVE('',#12068,#12066,#6206,.T.);
#16129=EDGE_CURVE('',#12069,#12067,#6207,.T.);
#16130=EDGE_CURVE('',#12068,#12069,#7716,.T.);
#16131=EDGE_CURVE('',#12070,#12068,#7717,.T.);
#16132=EDGE_CURVE('',#12071,#12069,#7718,.T.);
#16133=EDGE_CURVE('',#12070,#12071,#7719,.T.);
#16134=EDGE_CURVE('',#11889,#12070,#7720,.T.);
#16135=EDGE_CURVE('',#11890,#12071,#7721,.T.);
#22991=ORIENTED_EDGE('',*,*,#15857,.T.);
#22992=ORIENTED_EDGE('',*,*,#15858,.T.);
#22993=ORIENTED_EDGE('',*,*,#15859,.F.);
#22994=ORIENTED_EDGE('',*,*,#15858,.F.);
#22995=ORIENTED_EDGE('',*,*,#15860,.T.);
#22996=ORIENTED_EDGE('',*,*,#15861,.T.);
#22997=ORIENTED_EDGE('',*,*,#15862,.F.);
#22998=ORIENTED_EDGE('',*,*,#15863,.F.);
#22999=ORIENTED_EDGE('',*,*,#15864,.F.);
#23000=ORIENTED_EDGE('',*,*,#15863,.T.);
#23001=ORIENTED_EDGE('',*,*,#15865,.F.);
#23002=ORIENTED_EDGE('',*,*,#15866,.F.);
#23003=ORIENTED_EDGE('',*,*,#15867,.T.);
#23004=ORIENTED_EDGE('',*,*,#15866,.T.);
#23005=ORIENTED_EDGE('',*,*,#15868,.F.);
#23006=ORIENTED_EDGE('',*,*,#15869,.F.);
#23007=ORIENTED_EDGE('',*,*,#15870,.T.);
#23008=ORIENTED_EDGE('',*,*,#15869,.T.);
#23009=ORIENTED_EDGE('',*,*,#15871,.F.);
#23010=ORIENTED_EDGE('',*,*,#15872,.F.);
#23011=ORIENTED_EDGE('',*,*,#15873,.F.);
#23012=ORIENTED_EDGE('',*,*,#15872,.T.);
#23013=ORIENTED_EDGE('',*,*,#15874,.F.);
#23014=ORIENTED_EDGE('',*,*,#15875,.F.);
#23015=ORIENTED_EDGE('',*,*,#15876,.T.);
#23016=ORIENTED_EDGE('',*,*,#15875,.T.);
#23017=ORIENTED_EDGE('',*,*,#15877,.F.);
#23018=ORIENTED_EDGE('',*,*,#15878,.F.);
#23019=ORIENTED_EDGE('',*,*,#15879,.T.);
#23020=ORIENTED_EDGE('',*,*,#15878,.T.);
#23021=ORIENTED_EDGE('',*,*,#15880,.F.);
#23022=ORIENTED_EDGE('',*,*,#15881,.F.);
#23023=ORIENTED_EDGE('',*,*,#15882,.F.);
#23024=ORIENTED_EDGE('',*,*,#15881,.T.);
#23025=ORIENTED_EDGE('',*,*,#15883,.F.);
#23026=ORIENTED_EDGE('',*,*,#15884,.F.);
#23027=ORIENTED_EDGE('',*,*,#15885,.F.);
#23028=ORIENTED_EDGE('',*,*,#15884,.T.);
#23029=ORIENTED_EDGE('',*,*,#15886,.F.);
#23030=ORIENTED_EDGE('',*,*,#15887,.F.);
#23031=ORIENTED_EDGE('',*,*,#15888,.T.);
#23032=ORIENTED_EDGE('',*,*,#15887,.T.);
#23033=ORIENTED_EDGE('',*,*,#15889,.F.);
#23034=ORIENTED_EDGE('',*,*,#15890,.F.);
#23035=ORIENTED_EDGE('',*,*,#15891,.F.);
#23036=ORIENTED_EDGE('',*,*,#15890,.T.);
#23037=ORIENTED_EDGE('',*,*,#15892,.F.);
#23038=ORIENTED_EDGE('',*,*,#15893,.F.);
#23039=ORIENTED_EDGE('',*,*,#15894,.T.);
#23040=ORIENTED_EDGE('',*,*,#15893,.T.);
#23041=ORIENTED_EDGE('',*,*,#15895,.F.);
#23042=ORIENTED_EDGE('',*,*,#15896,.F.);
#23043=ORIENTED_EDGE('',*,*,#15897,.T.);
#23044=ORIENTED_EDGE('',*,*,#15896,.T.);
#23045=ORIENTED_EDGE('',*,*,#15898,.F.);
#23046=ORIENTED_EDGE('',*,*,#15899,.F.);
#23047=ORIENTED_EDGE('',*,*,#15900,.F.);
#23048=ORIENTED_EDGE('',*,*,#15899,.T.);
#23049=ORIENTED_EDGE('',*,*,#15901,.F.);
#23050=ORIENTED_EDGE('',*,*,#15902,.F.);
#23051=ORIENTED_EDGE('',*,*,#15903,.F.);
#23052=ORIENTED_EDGE('',*,*,#15902,.T.);
#23053=ORIENTED_EDGE('',*,*,#15904,.F.);
#23054=ORIENTED_EDGE('',*,*,#15905,.F.);
#23055=ORIENTED_EDGE('',*,*,#15906,.F.);
#23056=ORIENTED_EDGE('',*,*,#15905,.T.);
#23057=ORIENTED_EDGE('',*,*,#15907,.F.);
#23058=ORIENTED_EDGE('',*,*,#15908,.F.);
#23059=ORIENTED_EDGE('',*,*,#15909,.F.);
#23060=ORIENTED_EDGE('',*,*,#15908,.T.);
#23061=ORIENTED_EDGE('',*,*,#15910,.F.);
#23062=ORIENTED_EDGE('',*,*,#15911,.F.);
#23063=ORIENTED_EDGE('',*,*,#15912,.T.);
#23064=ORIENTED_EDGE('',*,*,#15911,.T.);
#23065=ORIENTED_EDGE('',*,*,#15913,.F.);
#23066=ORIENTED_EDGE('',*,*,#15914,.F.);
#23067=ORIENTED_EDGE('',*,*,#15915,.F.);
#23068=ORIENTED_EDGE('',*,*,#15914,.T.);
#23069=ORIENTED_EDGE('',*,*,#15916,.F.);
#23070=ORIENTED_EDGE('',*,*,#15917,.F.);
#23071=ORIENTED_EDGE('',*,*,#15918,.T.);
#23072=ORIENTED_EDGE('',*,*,#15917,.T.);
#23073=ORIENTED_EDGE('',*,*,#15919,.F.);
#23074=ORIENTED_EDGE('',*,*,#15920,.F.);
#23075=ORIENTED_EDGE('',*,*,#15921,.F.);
#23076=ORIENTED_EDGE('',*,*,#15920,.T.);
#23077=ORIENTED_EDGE('',*,*,#15922,.F.);
#23078=ORIENTED_EDGE('',*,*,#15923,.F.);
#23079=ORIENTED_EDGE('',*,*,#15924,.F.);
#23080=ORIENTED_EDGE('',*,*,#15923,.T.);
#23081=ORIENTED_EDGE('',*,*,#15925,.F.);
#23082=ORIENTED_EDGE('',*,*,#15926,.F.);
#23083=ORIENTED_EDGE('',*,*,#15927,.F.);
#23084=ORIENTED_EDGE('',*,*,#15926,.T.);
#23085=ORIENTED_EDGE('',*,*,#15928,.F.);
#23086=ORIENTED_EDGE('',*,*,#15929,.F.);
#23087=ORIENTED_EDGE('',*,*,#15930,.F.);
#23088=ORIENTED_EDGE('',*,*,#15929,.T.);
#23089=ORIENTED_EDGE('',*,*,#15931,.F.);
#23090=ORIENTED_EDGE('',*,*,#15932,.F.);
#23091=ORIENTED_EDGE('',*,*,#15933,.F.);
#23092=ORIENTED_EDGE('',*,*,#15932,.T.);
#23093=ORIENTED_EDGE('',*,*,#15934,.F.);
#23094=ORIENTED_EDGE('',*,*,#15935,.F.);
#23095=ORIENTED_EDGE('',*,*,#15936,.F.);
#23096=ORIENTED_EDGE('',*,*,#15935,.T.);
#23097=ORIENTED_EDGE('',*,*,#15937,.F.);
#23098=ORIENTED_EDGE('',*,*,#15938,.F.);
#23099=ORIENTED_EDGE('',*,*,#15939,.T.);
#23100=ORIENTED_EDGE('',*,*,#15938,.T.);
#23101=ORIENTED_EDGE('',*,*,#15940,.F.);
#23102=ORIENTED_EDGE('',*,*,#15941,.F.);
#23103=ORIENTED_EDGE('',*,*,#15942,.F.);
#23104=ORIENTED_EDGE('',*,*,#15941,.T.);
#23105=ORIENTED_EDGE('',*,*,#15943,.F.);
#23106=ORIENTED_EDGE('',*,*,#15944,.F.);
#23107=ORIENTED_EDGE('',*,*,#15945,.T.);
#23108=ORIENTED_EDGE('',*,*,#15944,.T.);
#23109=ORIENTED_EDGE('',*,*,#15946,.F.);
#23110=ORIENTED_EDGE('',*,*,#15947,.F.);
#23111=ORIENTED_EDGE('',*,*,#15948,.F.);
#23112=ORIENTED_EDGE('',*,*,#15947,.T.);
#23113=ORIENTED_EDGE('',*,*,#15949,.F.);
#23114=ORIENTED_EDGE('',*,*,#15950,.F.);
#23115=ORIENTED_EDGE('',*,*,#15951,.T.);
#23116=ORIENTED_EDGE('',*,*,#15950,.T.);
#23117=ORIENTED_EDGE('',*,*,#15952,.F.);
#23118=ORIENTED_EDGE('',*,*,#15953,.F.);
#23119=ORIENTED_EDGE('',*,*,#15954,.T.);
#23120=ORIENTED_EDGE('',*,*,#15953,.T.);
#23121=ORIENTED_EDGE('',*,*,#15955,.F.);
#23122=ORIENTED_EDGE('',*,*,#15956,.F.);
#23123=ORIENTED_EDGE('',*,*,#15957,.T.);
#23124=ORIENTED_EDGE('',*,*,#15956,.T.);
#23125=ORIENTED_EDGE('',*,*,#15958,.F.);
#23126=ORIENTED_EDGE('',*,*,#15959,.F.);
#23127=ORIENTED_EDGE('',*,*,#15960,.T.);
#23128=ORIENTED_EDGE('',*,*,#15959,.T.);
#23129=ORIENTED_EDGE('',*,*,#15961,.F.);
#23130=ORIENTED_EDGE('',*,*,#15962,.F.);
#23131=ORIENTED_EDGE('',*,*,#15963,.T.);
#23132=ORIENTED_EDGE('',*,*,#15962,.T.);
#23133=ORIENTED_EDGE('',*,*,#15964,.F.);
#23134=ORIENTED_EDGE('',*,*,#15965,.F.);
#23135=ORIENTED_EDGE('',*,*,#15966,.T.);
#23136=ORIENTED_EDGE('',*,*,#15965,.T.);
#23137=ORIENTED_EDGE('',*,*,#15967,.F.);
#23138=ORIENTED_EDGE('',*,*,#15968,.F.);
#23139=ORIENTED_EDGE('',*,*,#15969,.T.);
#23140=ORIENTED_EDGE('',*,*,#15968,.T.);
#23141=ORIENTED_EDGE('',*,*,#15970,.F.);
#23142=ORIENTED_EDGE('',*,*,#15971,.F.);
#23143=ORIENTED_EDGE('',*,*,#15972,.F.);
#23144=ORIENTED_EDGE('',*,*,#15971,.T.);
#23145=ORIENTED_EDGE('',*,*,#15973,.F.);
#23146=ORIENTED_EDGE('',*,*,#15974,.F.);
#23147=ORIENTED_EDGE('',*,*,#15975,.T.);
#23148=ORIENTED_EDGE('',*,*,#15974,.T.);
#23149=ORIENTED_EDGE('',*,*,#15976,.F.);
#23150=ORIENTED_EDGE('',*,*,#15977,.F.);
#23151=ORIENTED_EDGE('',*,*,#15978,.T.);
#23152=ORIENTED_EDGE('',*,*,#15977,.T.);
#23153=ORIENTED_EDGE('',*,*,#15979,.F.);
#23154=ORIENTED_EDGE('',*,*,#15980,.F.);
#23155=ORIENTED_EDGE('',*,*,#15981,.F.);
#23156=ORIENTED_EDGE('',*,*,#15980,.T.);
#23157=ORIENTED_EDGE('',*,*,#15982,.F.);
#23158=ORIENTED_EDGE('',*,*,#15983,.F.);
#23159=ORIENTED_EDGE('',*,*,#15984,.T.);
#23160=ORIENTED_EDGE('',*,*,#15983,.T.);
#23161=ORIENTED_EDGE('',*,*,#15985,.F.);
#23162=ORIENTED_EDGE('',*,*,#15986,.F.);
#23163=ORIENTED_EDGE('',*,*,#15987,.F.);
#23164=ORIENTED_EDGE('',*,*,#15986,.T.);
#23165=ORIENTED_EDGE('',*,*,#15988,.F.);
#23166=ORIENTED_EDGE('',*,*,#15989,.F.);
#23167=ORIENTED_EDGE('',*,*,#15990,.T.);
#23168=ORIENTED_EDGE('',*,*,#15989,.T.);
#23169=ORIENTED_EDGE('',*,*,#15991,.F.);
#23170=ORIENTED_EDGE('',*,*,#15992,.F.);
#23171=ORIENTED_EDGE('',*,*,#15993,.T.);
#23172=ORIENTED_EDGE('',*,*,#15992,.T.);
#23173=ORIENTED_EDGE('',*,*,#15994,.F.);
#23174=ORIENTED_EDGE('',*,*,#15995,.F.);
#23175=ORIENTED_EDGE('',*,*,#15996,.T.);
#23176=ORIENTED_EDGE('',*,*,#15995,.T.);
#23177=ORIENTED_EDGE('',*,*,#15997,.F.);
#23178=ORIENTED_EDGE('',*,*,#15998,.F.);
#23179=ORIENTED_EDGE('',*,*,#15999,.T.);
#23180=ORIENTED_EDGE('',*,*,#15998,.T.);
#23181=ORIENTED_EDGE('',*,*,#16000,.F.);
#23182=ORIENTED_EDGE('',*,*,#16001,.F.);
#23183=ORIENTED_EDGE('',*,*,#16002,.T.);
#23184=ORIENTED_EDGE('',*,*,#16001,.T.);
#23185=ORIENTED_EDGE('',*,*,#16003,.F.);
#23186=ORIENTED_EDGE('',*,*,#16004,.F.);
#23187=ORIENTED_EDGE('',*,*,#16005,.T.);
#23188=ORIENTED_EDGE('',*,*,#16004,.T.);
#23189=ORIENTED_EDGE('',*,*,#16006,.F.);
#23190=ORIENTED_EDGE('',*,*,#16007,.F.);
#23191=ORIENTED_EDGE('',*,*,#16008,.F.);
#23192=ORIENTED_EDGE('',*,*,#16007,.T.);
#23193=ORIENTED_EDGE('',*,*,#16009,.F.);
#23194=ORIENTED_EDGE('',*,*,#16010,.F.);
#23195=ORIENTED_EDGE('',*,*,#16011,.F.);
#23196=ORIENTED_EDGE('',*,*,#16010,.T.);
#23197=ORIENTED_EDGE('',*,*,#16012,.F.);
#23198=ORIENTED_EDGE('',*,*,#16013,.F.);
#23199=ORIENTED_EDGE('',*,*,#16014,.F.);
#23200=ORIENTED_EDGE('',*,*,#16013,.T.);
#23201=ORIENTED_EDGE('',*,*,#16015,.F.);
#23202=ORIENTED_EDGE('',*,*,#16016,.F.);
#23203=ORIENTED_EDGE('',*,*,#16017,.T.);
#23204=ORIENTED_EDGE('',*,*,#16016,.T.);
#23205=ORIENTED_EDGE('',*,*,#16018,.F.);
#23206=ORIENTED_EDGE('',*,*,#16019,.F.);
#23207=ORIENTED_EDGE('',*,*,#16020,.F.);
#23208=ORIENTED_EDGE('',*,*,#16019,.T.);
#23209=ORIENTED_EDGE('',*,*,#16021,.F.);
#23210=ORIENTED_EDGE('',*,*,#16022,.F.);
#23211=ORIENTED_EDGE('',*,*,#16023,.F.);
#23212=ORIENTED_EDGE('',*,*,#16022,.T.);
#23213=ORIENTED_EDGE('',*,*,#16024,.F.);
#23214=ORIENTED_EDGE('',*,*,#16025,.F.);
#23215=ORIENTED_EDGE('',*,*,#16026,.T.);
#23216=ORIENTED_EDGE('',*,*,#16025,.T.);
#23217=ORIENTED_EDGE('',*,*,#16027,.F.);
#23218=ORIENTED_EDGE('',*,*,#16028,.F.);
#23219=ORIENTED_EDGE('',*,*,#16029,.F.);
#23220=ORIENTED_EDGE('',*,*,#16028,.T.);
#23221=ORIENTED_EDGE('',*,*,#16030,.F.);
#23222=ORIENTED_EDGE('',*,*,#16031,.F.);
#23223=ORIENTED_EDGE('',*,*,#16032,.T.);
#23224=ORIENTED_EDGE('',*,*,#16031,.T.);
#23225=ORIENTED_EDGE('',*,*,#16033,.F.);
#23226=ORIENTED_EDGE('',*,*,#16034,.F.);
#23227=ORIENTED_EDGE('',*,*,#16035,.T.);
#23228=ORIENTED_EDGE('',*,*,#16034,.T.);
#23229=ORIENTED_EDGE('',*,*,#16036,.F.);
#23230=ORIENTED_EDGE('',*,*,#16037,.F.);
#23231=ORIENTED_EDGE('',*,*,#16038,.F.);
#23232=ORIENTED_EDGE('',*,*,#16037,.T.);
#23233=ORIENTED_EDGE('',*,*,#16039,.F.);
#23234=ORIENTED_EDGE('',*,*,#16040,.F.);
#23235=ORIENTED_EDGE('',*,*,#16041,.F.);
#23236=ORIENTED_EDGE('',*,*,#16040,.T.);
#23237=ORIENTED_EDGE('',*,*,#16042,.F.);
#23238=ORIENTED_EDGE('',*,*,#16043,.F.);
#23239=ORIENTED_EDGE('',*,*,#16044,.F.);
#23240=ORIENTED_EDGE('',*,*,#16043,.T.);
#23241=ORIENTED_EDGE('',*,*,#16045,.F.);
#23242=ORIENTED_EDGE('',*,*,#16046,.F.);
#23243=ORIENTED_EDGE('',*,*,#16047,.F.);
#23244=ORIENTED_EDGE('',*,*,#16046,.T.);
#23245=ORIENTED_EDGE('',*,*,#16048,.F.);
#23246=ORIENTED_EDGE('',*,*,#16049,.F.);
#23247=ORIENTED_EDGE('',*,*,#16050,.T.);
#23248=ORIENTED_EDGE('',*,*,#16049,.T.);
#23249=ORIENTED_EDGE('',*,*,#16051,.F.);
#23250=ORIENTED_EDGE('',*,*,#16052,.F.);
#23251=ORIENTED_EDGE('',*,*,#16053,.F.);
#23252=ORIENTED_EDGE('',*,*,#16052,.T.);
#23253=ORIENTED_EDGE('',*,*,#16054,.F.);
#23254=ORIENTED_EDGE('',*,*,#16055,.F.);
#23255=ORIENTED_EDGE('',*,*,#16056,.T.);
#23256=ORIENTED_EDGE('',*,*,#16055,.T.);
#23257=ORIENTED_EDGE('',*,*,#16057,.F.);
#23258=ORIENTED_EDGE('',*,*,#16058,.F.);
#23259=ORIENTED_EDGE('',*,*,#16059,.F.);
#23260=ORIENTED_EDGE('',*,*,#16058,.T.);
#23261=ORIENTED_EDGE('',*,*,#16060,.F.);
#23262=ORIENTED_EDGE('',*,*,#16061,.F.);
#23263=ORIENTED_EDGE('',*,*,#16062,.F.);
#23264=ORIENTED_EDGE('',*,*,#16061,.T.);
#23265=ORIENTED_EDGE('',*,*,#16063,.F.);
#23266=ORIENTED_EDGE('',*,*,#16064,.F.);
#23267=ORIENTED_EDGE('',*,*,#16065,.F.);
#23268=ORIENTED_EDGE('',*,*,#16064,.T.);
#23269=ORIENTED_EDGE('',*,*,#16066,.F.);
#23270=ORIENTED_EDGE('',*,*,#16067,.F.);
#23271=ORIENTED_EDGE('',*,*,#16068,.F.);
#23272=ORIENTED_EDGE('',*,*,#16067,.T.);
#23273=ORIENTED_EDGE('',*,*,#16069,.F.);
#23274=ORIENTED_EDGE('',*,*,#16070,.F.);
#23275=ORIENTED_EDGE('',*,*,#16071,.F.);
#23276=ORIENTED_EDGE('',*,*,#16070,.T.);
#23277=ORIENTED_EDGE('',*,*,#16072,.F.);
#23278=ORIENTED_EDGE('',*,*,#16073,.F.);
#23279=ORIENTED_EDGE('',*,*,#16074,.F.);
#23280=ORIENTED_EDGE('',*,*,#16073,.T.);
#23281=ORIENTED_EDGE('',*,*,#16075,.F.);
#23282=ORIENTED_EDGE('',*,*,#16076,.F.);
#23283=ORIENTED_EDGE('',*,*,#16077,.F.);
#23284=ORIENTED_EDGE('',*,*,#16076,.T.);
#23285=ORIENTED_EDGE('',*,*,#16078,.F.);
#23286=ORIENTED_EDGE('',*,*,#16079,.F.);
#23287=ORIENTED_EDGE('',*,*,#16080,.F.);
#23288=ORIENTED_EDGE('',*,*,#16079,.T.);
#23289=ORIENTED_EDGE('',*,*,#16081,.F.);
#23290=ORIENTED_EDGE('',*,*,#16082,.F.);
#23291=ORIENTED_EDGE('',*,*,#16083,.T.);
#23292=ORIENTED_EDGE('',*,*,#16082,.T.);
#23293=ORIENTED_EDGE('',*,*,#16084,.F.);
#23294=ORIENTED_EDGE('',*,*,#16085,.F.);
#23295=ORIENTED_EDGE('',*,*,#16086,.F.);
#23296=ORIENTED_EDGE('',*,*,#16085,.T.);
#23297=ORIENTED_EDGE('',*,*,#16087,.F.);
#23298=ORIENTED_EDGE('',*,*,#16088,.F.);
#23299=ORIENTED_EDGE('',*,*,#16089,.T.);
#23300=ORIENTED_EDGE('',*,*,#16088,.T.);
#23301=ORIENTED_EDGE('',*,*,#16090,.F.);
#23302=ORIENTED_EDGE('',*,*,#16091,.F.);
#23303=ORIENTED_EDGE('',*,*,#16092,.T.);
#23304=ORIENTED_EDGE('',*,*,#16091,.T.);
#23305=ORIENTED_EDGE('',*,*,#16093,.F.);
#23306=ORIENTED_EDGE('',*,*,#16094,.F.);
#23307=ORIENTED_EDGE('',*,*,#16095,.T.);
#23308=ORIENTED_EDGE('',*,*,#16094,.T.);
#23309=ORIENTED_EDGE('',*,*,#16096,.F.);
#23310=ORIENTED_EDGE('',*,*,#16097,.F.);
#23311=ORIENTED_EDGE('',*,*,#16098,.T.);
#23312=ORIENTED_EDGE('',*,*,#16097,.T.);
#23313=ORIENTED_EDGE('',*,*,#16099,.F.);
#23314=ORIENTED_EDGE('',*,*,#16100,.F.);
#23315=ORIENTED_EDGE('',*,*,#16101,.T.);
#23316=ORIENTED_EDGE('',*,*,#16100,.T.);
#23317=ORIENTED_EDGE('',*,*,#16102,.F.);
#23318=ORIENTED_EDGE('',*,*,#16103,.F.);
#23319=ORIENTED_EDGE('',*,*,#16104,.T.);
#23320=ORIENTED_EDGE('',*,*,#16103,.T.);
#23321=ORIENTED_EDGE('',*,*,#16105,.F.);
#23322=ORIENTED_EDGE('',*,*,#16106,.F.);
#23323=ORIENTED_EDGE('',*,*,#16107,.T.);
#23324=ORIENTED_EDGE('',*,*,#16106,.T.);
#23325=ORIENTED_EDGE('',*,*,#16108,.F.);
#23326=ORIENTED_EDGE('',*,*,#16109,.F.);
#23327=ORIENTED_EDGE('',*,*,#16110,.F.);
#23328=ORIENTED_EDGE('',*,*,#16109,.T.);
#23329=ORIENTED_EDGE('',*,*,#16111,.F.);
#23330=ORIENTED_EDGE('',*,*,#16112,.F.);
#23331=ORIENTED_EDGE('',*,*,#16113,.T.);
#23332=ORIENTED_EDGE('',*,*,#16112,.T.);
#23333=ORIENTED_EDGE('',*,*,#16114,.F.);
#23334=ORIENTED_EDGE('',*,*,#16115,.F.);
#23335=ORIENTED_EDGE('',*,*,#16116,.T.);
#23336=ORIENTED_EDGE('',*,*,#16115,.T.);
#23337=ORIENTED_EDGE('',*,*,#16117,.F.);
#23338=ORIENTED_EDGE('',*,*,#16118,.F.);
#23339=ORIENTED_EDGE('',*,*,#16119,.F.);
#23340=ORIENTED_EDGE('',*,*,#16118,.T.);
#23341=ORIENTED_EDGE('',*,*,#16120,.F.);
#23342=ORIENTED_EDGE('',*,*,#16121,.F.);
#23343=ORIENTED_EDGE('',*,*,#16122,.T.);
#23344=ORIENTED_EDGE('',*,*,#16121,.T.);
#23345=ORIENTED_EDGE('',*,*,#16123,.F.);
#23346=ORIENTED_EDGE('',*,*,#16124,.F.);
#23347=ORIENTED_EDGE('',*,*,#16125,.F.);
#23348=ORIENTED_EDGE('',*,*,#16124,.T.);
#23349=ORIENTED_EDGE('',*,*,#16126,.F.);
#23350=ORIENTED_EDGE('',*,*,#16127,.F.);
#23351=ORIENTED_EDGE('',*,*,#16128,.T.);
#23352=ORIENTED_EDGE('',*,*,#16127,.T.);
#23353=ORIENTED_EDGE('',*,*,#16129,.F.);
#23354=ORIENTED_EDGE('',*,*,#16130,.F.);
#23355=ORIENTED_EDGE('',*,*,#16131,.T.);
#23356=ORIENTED_EDGE('',*,*,#16130,.T.);
#23357=ORIENTED_EDGE('',*,*,#16132,.F.);
#23358=ORIENTED_EDGE('',*,*,#16133,.F.);
#23359=ORIENTED_EDGE('',*,*,#16134,.T.);
#23360=ORIENTED_EDGE('',*,*,#16133,.T.);
#23361=ORIENTED_EDGE('',*,*,#16135,.F.);
#23362=ORIENTED_EDGE('',*,*,#15861,.F.);
#23363=ORIENTED_EDGE('',*,*,#16135,.T.);
#23364=ORIENTED_EDGE('',*,*,#16132,.T.);
#23365=ORIENTED_EDGE('',*,*,#16129,.T.);
#23366=ORIENTED_EDGE('',*,*,#16126,.T.);
#23367=ORIENTED_EDGE('',*,*,#16123,.T.);
#23368=ORIENTED_EDGE('',*,*,#16120,.T.);
#23369=ORIENTED_EDGE('',*,*,#16117,.T.);
#23370=ORIENTED_EDGE('',*,*,#16114,.T.);
#23371=ORIENTED_EDGE('',*,*,#16111,.T.);
#23372=ORIENTED_EDGE('',*,*,#16108,.T.);
#23373=ORIENTED_EDGE('',*,*,#16105,.T.);
#23374=ORIENTED_EDGE('',*,*,#16102,.T.);
#23375=ORIENTED_EDGE('',*,*,#16099,.T.);
#23376=ORIENTED_EDGE('',*,*,#16096,.T.);
#23377=ORIENTED_EDGE('',*,*,#16093,.T.);
#23378=ORIENTED_EDGE('',*,*,#16090,.T.);
#23379=ORIENTED_EDGE('',*,*,#16087,.T.);
#23380=ORIENTED_EDGE('',*,*,#16084,.T.);
#23381=ORIENTED_EDGE('',*,*,#16081,.T.);
#23382=ORIENTED_EDGE('',*,*,#16078,.T.);
#23383=ORIENTED_EDGE('',*,*,#16075,.T.);
#23384=ORIENTED_EDGE('',*,*,#16072,.T.);
#23385=ORIENTED_EDGE('',*,*,#16069,.T.);
#23386=ORIENTED_EDGE('',*,*,#16066,.T.);
#23387=ORIENTED_EDGE('',*,*,#16063,.T.);
#23388=ORIENTED_EDGE('',*,*,#16060,.T.);
#23389=ORIENTED_EDGE('',*,*,#16057,.T.);
#23390=ORIENTED_EDGE('',*,*,#16054,.T.);
#23391=ORIENTED_EDGE('',*,*,#16051,.T.);
#23392=ORIENTED_EDGE('',*,*,#16048,.T.);
#23393=ORIENTED_EDGE('',*,*,#16045,.T.);
#23394=ORIENTED_EDGE('',*,*,#16042,.T.);
#23395=ORIENTED_EDGE('',*,*,#16039,.T.);
#23396=ORIENTED_EDGE('',*,*,#16036,.T.);
#23397=ORIENTED_EDGE('',*,*,#16033,.T.);
#23398=ORIENTED_EDGE('',*,*,#16030,.T.);
#23399=ORIENTED_EDGE('',*,*,#16027,.T.);
#23400=ORIENTED_EDGE('',*,*,#16024,.T.);
#23401=ORIENTED_EDGE('',*,*,#16021,.T.);
#23402=ORIENTED_EDGE('',*,*,#16018,.T.);
#23403=ORIENTED_EDGE('',*,*,#16015,.T.);
#23404=ORIENTED_EDGE('',*,*,#16012,.T.);
#23405=ORIENTED_EDGE('',*,*,#16009,.T.);
#23406=ORIENTED_EDGE('',*,*,#16006,.T.);
#23407=ORIENTED_EDGE('',*,*,#16003,.T.);
#23408=ORIENTED_EDGE('',*,*,#16000,.T.);
#23409=ORIENTED_EDGE('',*,*,#15997,.T.);
#23410=ORIENTED_EDGE('',*,*,#15994,.T.);
#23411=ORIENTED_EDGE('',*,*,#15991,.T.);
#23412=ORIENTED_EDGE('',*,*,#15988,.T.);
#23413=ORIENTED_EDGE('',*,*,#15985,.T.);
#23414=ORIENTED_EDGE('',*,*,#15982,.T.);
#23415=ORIENTED_EDGE('',*,*,#15979,.T.);
#23416=ORIENTED_EDGE('',*,*,#15976,.T.);
#23417=ORIENTED_EDGE('',*,*,#15973,.T.);
#23418=ORIENTED_EDGE('',*,*,#15970,.T.);
#23419=ORIENTED_EDGE('',*,*,#15967,.T.);
#23420=ORIENTED_EDGE('',*,*,#15964,.T.);
#23421=ORIENTED_EDGE('',*,*,#15961,.T.);
#23422=ORIENTED_EDGE('',*,*,#15958,.T.);
#23423=ORIENTED_EDGE('',*,*,#15955,.T.);
#23424=ORIENTED_EDGE('',*,*,#15952,.T.);
#23425=ORIENTED_EDGE('',*,*,#15949,.T.);
#23426=ORIENTED_EDGE('',*,*,#15946,.T.);
#23427=ORIENTED_EDGE('',*,*,#15943,.T.);
#23428=ORIENTED_EDGE('',*,*,#15940,.T.);
#23429=ORIENTED_EDGE('',*,*,#15937,.T.);
#23430=ORIENTED_EDGE('',*,*,#15934,.T.);
#23431=ORIENTED_EDGE('',*,*,#15931,.T.);
#23432=ORIENTED_EDGE('',*,*,#15928,.T.);
#23433=ORIENTED_EDGE('',*,*,#15925,.T.);
#23434=ORIENTED_EDGE('',*,*,#15922,.T.);
#23435=ORIENTED_EDGE('',*,*,#15919,.T.);
#23436=ORIENTED_EDGE('',*,*,#15916,.T.);
#23437=ORIENTED_EDGE('',*,*,#15913,.T.);
#23438=ORIENTED_EDGE('',*,*,#15910,.T.);
#23439=ORIENTED_EDGE('',*,*,#15907,.T.);
#23440=ORIENTED_EDGE('',*,*,#15904,.T.);
#23441=ORIENTED_EDGE('',*,*,#15901,.T.);
#23442=ORIENTED_EDGE('',*,*,#15898,.T.);
#23443=ORIENTED_EDGE('',*,*,#15895,.T.);
#23444=ORIENTED_EDGE('',*,*,#15892,.T.);
#23445=ORIENTED_EDGE('',*,*,#15889,.T.);
#23446=ORIENTED_EDGE('',*,*,#15886,.T.);
#23447=ORIENTED_EDGE('',*,*,#15883,.T.);
#23448=ORIENTED_EDGE('',*,*,#15880,.T.);
#23449=ORIENTED_EDGE('',*,*,#15877,.T.);
#23450=ORIENTED_EDGE('',*,*,#15874,.T.);
#23451=ORIENTED_EDGE('',*,*,#15871,.T.);
#23452=ORIENTED_EDGE('',*,*,#15868,.T.);
#23453=ORIENTED_EDGE('',*,*,#15865,.T.);
#23454=ORIENTED_EDGE('',*,*,#15862,.T.);
#23455=ORIENTED_EDGE('',*,*,#15859,.T.);
#23456=ORIENTED_EDGE('',*,*,#16134,.F.);
#23457=ORIENTED_EDGE('',*,*,#15860,.F.);
#23458=ORIENTED_EDGE('',*,*,#15864,.T.);
#23459=ORIENTED_EDGE('',*,*,#15867,.F.);
#23460=ORIENTED_EDGE('',*,*,#15870,.F.);
#23461=ORIENTED_EDGE('',*,*,#15873,.T.);
#23462=ORIENTED_EDGE('',*,*,#15876,.F.);
#23463=ORIENTED_EDGE('',*,*,#15879,.F.);
#23464=ORIENTED_EDGE('',*,*,#15882,.T.);
#23465=ORIENTED_EDGE('',*,*,#15885,.T.);
#23466=ORIENTED_EDGE('',*,*,#15888,.F.);
#23467=ORIENTED_EDGE('',*,*,#15891,.T.);
#23468=ORIENTED_EDGE('',*,*,#15894,.F.);
#23469=ORIENTED_EDGE('',*,*,#15897,.F.);
#23470=ORIENTED_EDGE('',*,*,#15900,.T.);
#23471=ORIENTED_EDGE('',*,*,#15903,.T.);
#23472=ORIENTED_EDGE('',*,*,#15906,.T.);
#23473=ORIENTED_EDGE('',*,*,#15909,.T.);
#23474=ORIENTED_EDGE('',*,*,#15912,.F.);
#23475=ORIENTED_EDGE('',*,*,#15915,.T.);
#23476=ORIENTED_EDGE('',*,*,#15918,.F.);
#23477=ORIENTED_EDGE('',*,*,#15921,.T.);
#23478=ORIENTED_EDGE('',*,*,#15924,.T.);
#23479=ORIENTED_EDGE('',*,*,#15927,.T.);
#23480=ORIENTED_EDGE('',*,*,#15930,.T.);
#23481=ORIENTED_EDGE('',*,*,#15933,.T.);
#23482=ORIENTED_EDGE('',*,*,#15936,.T.);
#23483=ORIENTED_EDGE('',*,*,#15939,.F.);
#23484=ORIENTED_EDGE('',*,*,#15942,.T.);
#23485=ORIENTED_EDGE('',*,*,#15945,.F.);
#23486=ORIENTED_EDGE('',*,*,#15948,.T.);
#23487=ORIENTED_EDGE('',*,*,#15951,.F.);
#23488=ORIENTED_EDGE('',*,*,#15954,.F.);
#23489=ORIENTED_EDGE('',*,*,#15957,.F.);
#23490=ORIENTED_EDGE('',*,*,#15960,.F.);
#23491=ORIENTED_EDGE('',*,*,#15963,.F.);
#23492=ORIENTED_EDGE('',*,*,#15966,.F.);
#23493=ORIENTED_EDGE('',*,*,#15969,.F.);
#23494=ORIENTED_EDGE('',*,*,#15972,.T.);
#23495=ORIENTED_EDGE('',*,*,#15975,.F.);
#23496=ORIENTED_EDGE('',*,*,#15978,.F.);
#23497=ORIENTED_EDGE('',*,*,#15981,.T.);
#23498=ORIENTED_EDGE('',*,*,#15984,.F.);
#23499=ORIENTED_EDGE('',*,*,#15987,.T.);
#23500=ORIENTED_EDGE('',*,*,#15990,.F.);
#23501=ORIENTED_EDGE('',*,*,#15993,.F.);
#23502=ORIENTED_EDGE('',*,*,#15996,.F.);
#23503=ORIENTED_EDGE('',*,*,#15999,.F.);
#23504=ORIENTED_EDGE('',*,*,#16002,.F.);
#23505=ORIENTED_EDGE('',*,*,#16005,.F.);
#23506=ORIENTED_EDGE('',*,*,#16008,.T.);
#23507=ORIENTED_EDGE('',*,*,#16011,.T.);
#23508=ORIENTED_EDGE('',*,*,#16014,.T.);
#23509=ORIENTED_EDGE('',*,*,#16017,.F.);
#23510=ORIENTED_EDGE('',*,*,#16020,.T.);
#23511=ORIENTED_EDGE('',*,*,#16023,.T.);
#23512=ORIENTED_EDGE('',*,*,#16026,.F.);
#23513=ORIENTED_EDGE('',*,*,#16029,.T.);
#23514=ORIENTED_EDGE('',*,*,#16032,.F.);
#23515=ORIENTED_EDGE('',*,*,#16035,.F.);
#23516=ORIENTED_EDGE('',*,*,#16038,.T.);
#23517=ORIENTED_EDGE('',*,*,#16041,.T.);
#23518=ORIENTED_EDGE('',*,*,#16044,.T.);
#23519=ORIENTED_EDGE('',*,*,#16047,.T.);
#23520=ORIENTED_EDGE('',*,*,#16050,.F.);
#23521=ORIENTED_EDGE('',*,*,#16053,.T.);
#23522=ORIENTED_EDGE('',*,*,#16056,.F.);
#23523=ORIENTED_EDGE('',*,*,#16059,.T.);
#23524=ORIENTED_EDGE('',*,*,#16062,.T.);
#23525=ORIENTED_EDGE('',*,*,#16065,.T.);
#23526=ORIENTED_EDGE('',*,*,#16068,.T.);
#23527=ORIENTED_EDGE('',*,*,#16071,.T.);
#23528=ORIENTED_EDGE('',*,*,#16074,.T.);
#23529=ORIENTED_EDGE('',*,*,#16077,.T.);
#23530=ORIENTED_EDGE('',*,*,#16080,.T.);
#23531=ORIENTED_EDGE('',*,*,#16083,.F.);
#23532=ORIENTED_EDGE('',*,*,#16086,.T.);
#23533=ORIENTED_EDGE('',*,*,#16089,.F.);
#23534=ORIENTED_EDGE('',*,*,#16092,.F.);
#23535=ORIENTED_EDGE('',*,*,#16095,.F.);
#23536=ORIENTED_EDGE('',*,*,#16098,.F.);
#23537=ORIENTED_EDGE('',*,*,#16101,.F.);
#23538=ORIENTED_EDGE('',*,*,#16104,.F.);
#23539=ORIENTED_EDGE('',*,*,#16107,.F.);
#23540=ORIENTED_EDGE('',*,*,#16110,.T.);
#23541=ORIENTED_EDGE('',*,*,#16113,.F.);
#23542=ORIENTED_EDGE('',*,*,#16116,.F.);
#23543=ORIENTED_EDGE('',*,*,#16119,.T.);
#23544=ORIENTED_EDGE('',*,*,#16122,.F.);
#23545=ORIENTED_EDGE('',*,*,#16125,.T.);
#23546=ORIENTED_EDGE('',*,*,#16128,.F.);
#23547=ORIENTED_EDGE('',*,*,#16131,.F.);
#23548=ORIENTED_EDGE('',*,*,#15857,.F.);
#26636=PLANE('',#29557);
#26637=PLANE('',#29558);
#26638=PLANE('',#29559);
#26639=PLANE('',#29560);
#26640=PLANE('',#29561);
#26641=PLANE('',#29565);
#26642=PLANE('',#29566);
#26643=PLANE('',#29576);
#26644=PLANE('',#29577);
#26645=PLANE('',#29578);
#26646=PLANE('',#29582);
#26647=PLANE('',#29586);
#26648=PLANE('',#29590);
#26649=PLANE('',#29591);
#26650=PLANE('',#29592);
#26651=PLANE('',#29596);
#26652=PLANE('',#29600);
#26653=PLANE('',#29604);
#26654=PLANE('',#29608);
#26655=PLANE('',#29609);
#26656=PLANE('',#29610);
#26657=PLANE('',#29614);
#26658=PLANE('',#29618);
#26659=PLANE('',#29622);
#26660=PLANE('',#29623);
#26661=PLANE('',#29624);
#26662=PLANE('',#29634);
#26663=PLANE('',#29635);
#26664=PLANE('',#29639);
#26665=PLANE('',#29640);
#26666=PLANE('',#29641);
#26667=PLANE('',#29642);
#26668=PLANE('',#29643);
#26669=PLANE('',#29647);
#26670=PLANE('',#29648);
#26671=PLANE('',#29658);
#26672=PLANE('',#29659);
#26673=PLANE('',#29660);
#26674=PLANE('',#29664);
#26675=PLANE('',#29668);
#26676=PLANE('',#29672);
#26677=PLANE('',#29673);
#26678=PLANE('',#29674);
#26679=PLANE('',#29678);
#26680=PLANE('',#29682);
#26681=PLANE('',#29686);
#26682=PLANE('',#29690);
#26683=PLANE('',#29691);
#26684=PLANE('',#29692);
#26685=PLANE('',#29696);
#26686=PLANE('',#29700);
#26687=PLANE('',#29704);
#26688=PLANE('',#29705);
#26689=PLANE('',#29706);
#26690=PLANE('',#29716);
#26691=PLANE('',#29717);
#26692=PLANE('',#29718);
#26693=PLANE('',#29719);
#27625=ADVANCED_FACE('',(#3822),#2652,.F.);
#27626=ADVANCED_FACE('',(#3823),#2653,.T.);
#27627=ADVANCED_FACE('',(#3824),#26636,.T.);
#27628=ADVANCED_FACE('',(#3825),#26637,.T.);
#27629=ADVANCED_FACE('',(#3826),#26638,.T.);
#27630=ADVANCED_FACE('',(#3827),#26639,.T.);
#27631=ADVANCED_FACE('',(#3828),#26640,.T.);
#27632=ADVANCED_FACE('',(#3829),#2654,.T.);
#27633=ADVANCED_FACE('',(#3830),#26641,.T.);
#27634=ADVANCED_FACE('',(#3831),#26642,.T.);
#27635=ADVANCED_FACE('',(#3832),#2655,.T.);
#27636=ADVANCED_FACE('',(#3833),#2656,.F.);
#27637=ADVANCED_FACE('',(#3834),#2657,.T.);
#27638=ADVANCED_FACE('',(#3835),#26643,.T.);
#27639=ADVANCED_FACE('',(#3836),#26644,.T.);
#27640=ADVANCED_FACE('',(#3837),#26645,.T.);
#27641=ADVANCED_FACE('',(#3838),#2658,.F.);
#27642=ADVANCED_FACE('',(#3839),#26646,.T.);
#27643=ADVANCED_FACE('',(#3840),#2659,.T.);
#27644=ADVANCED_FACE('',(#3841),#26647,.T.);
#27645=ADVANCED_FACE('',(#3842),#2660,.T.);
#27646=ADVANCED_FACE('',(#3843),#26648,.T.);
#27647=ADVANCED_FACE('',(#3844),#26649,.T.);
#27648=ADVANCED_FACE('',(#3845),#26650,.T.);
#27649=ADVANCED_FACE('',(#3846),#2661,.F.);
#27650=ADVANCED_FACE('',(#3847),#26651,.T.);
#27651=ADVANCED_FACE('',(#3848),#2662,.F.);
#27652=ADVANCED_FACE('',(#3849),#26652,.T.);
#27653=ADVANCED_FACE('',(#3850),#2663,.F.);
#27654=ADVANCED_FACE('',(#3851),#26653,.T.);
#27655=ADVANCED_FACE('',(#3852),#2664,.F.);
#27656=ADVANCED_FACE('',(#3853),#26654,.T.);
#27657=ADVANCED_FACE('',(#3854),#26655,.T.);
#27658=ADVANCED_FACE('',(#3855),#26656,.T.);
#27659=ADVANCED_FACE('',(#3856),#2665,.T.);
#27660=ADVANCED_FACE('',(#3857),#26657,.T.);
#27661=ADVANCED_FACE('',(#3858),#2666,.T.);
#27662=ADVANCED_FACE('',(#3859),#26658,.T.);
#27663=ADVANCED_FACE('',(#3860),#2667,.F.);
#27664=ADVANCED_FACE('',(#3861),#26659,.T.);
#27665=ADVANCED_FACE('',(#3862),#26660,.T.);
#27666=ADVANCED_FACE('',(#3863),#26661,.T.);
#27667=ADVANCED_FACE('',(#3864),#2668,.T.);
#27668=ADVANCED_FACE('',(#3865),#2669,.F.);
#27669=ADVANCED_FACE('',(#3866),#2670,.T.);
#27670=ADVANCED_FACE('',(#3867),#26662,.T.);
#27671=ADVANCED_FACE('',(#3868),#26663,.T.);
#27672=ADVANCED_FACE('',(#3869),#2671,.T.);
#27673=ADVANCED_FACE('',(#3870),#26664,.T.);
#27674=ADVANCED_FACE('',(#3871),#26665,.T.);
#27675=ADVANCED_FACE('',(#3872),#26666,.T.);
#27676=ADVANCED_FACE('',(#3873),#26667,.T.);
#27677=ADVANCED_FACE('',(#3874),#26668,.T.);
#27678=ADVANCED_FACE('',(#3875),#2672,.T.);
#27679=ADVANCED_FACE('',(#3876),#26669,.T.);
#27680=ADVANCED_FACE('',(#3877),#26670,.T.);
#27681=ADVANCED_FACE('',(#3878),#2673,.T.);
#27682=ADVANCED_FACE('',(#3879),#2674,.F.);
#27683=ADVANCED_FACE('',(#3880),#2675,.T.);
#27684=ADVANCED_FACE('',(#3881),#26671,.T.);
#27685=ADVANCED_FACE('',(#3882),#26672,.T.);
#27686=ADVANCED_FACE('',(#3883),#26673,.T.);
#27687=ADVANCED_FACE('',(#3884),#2676,.F.);
#27688=ADVANCED_FACE('',(#3885),#26674,.T.);
#27689=ADVANCED_FACE('',(#3886),#2677,.T.);
#27690=ADVANCED_FACE('',(#3887),#26675,.T.);
#27691=ADVANCED_FACE('',(#3888),#2678,.T.);
#27692=ADVANCED_FACE('',(#3889),#26676,.T.);
#27693=ADVANCED_FACE('',(#3890),#26677,.T.);
#27694=ADVANCED_FACE('',(#3891),#26678,.T.);
#27695=ADVANCED_FACE('',(#3892),#2679,.F.);
#27696=ADVANCED_FACE('',(#3893),#26679,.T.);
#27697=ADVANCED_FACE('',(#3894),#2680,.F.);
#27698=ADVANCED_FACE('',(#3895),#26680,.T.);
#27699=ADVANCED_FACE('',(#3896),#2681,.F.);
#27700=ADVANCED_FACE('',(#3897),#26681,.T.);
#27701=ADVANCED_FACE('',(#3898),#2682,.F.);
#27702=ADVANCED_FACE('',(#3899),#26682,.T.);
#27703=ADVANCED_FACE('',(#3900),#26683,.T.);
#27704=ADVANCED_FACE('',(#3901),#26684,.T.);
#27705=ADVANCED_FACE('',(#3902),#2683,.T.);
#27706=ADVANCED_FACE('',(#3903),#26685,.T.);
#27707=ADVANCED_FACE('',(#3904),#2684,.T.);
#27708=ADVANCED_FACE('',(#3905),#26686,.T.);
#27709=ADVANCED_FACE('',(#3906),#2685,.F.);
#27710=ADVANCED_FACE('',(#3907),#26687,.T.);
#27711=ADVANCED_FACE('',(#3908),#26688,.T.);
#27712=ADVANCED_FACE('',(#3909),#26689,.T.);
#27713=ADVANCED_FACE('',(#3910),#2686,.T.);
#27714=ADVANCED_FACE('',(#3911),#2687,.F.);
#27715=ADVANCED_FACE('',(#3912),#2688,.T.);
#27716=ADVANCED_FACE('',(#3913),#26690,.T.);
#27717=ADVANCED_FACE('',(#3914),#26691,.T.);
#27718=ADVANCED_FACE('',(#3915,#218),#26692,.T.);
#27719=ADVANCED_FACE('',(#3916,#219),#26693,.F.);
#28087=CLOSED_SHELL('',(#27625,#27626,#27627,#27628,#27629,#27630,#27631,
#27632,#27633,#27634,#27635,#27636,#27637,#27638,#27639,#27640,#27641,#27642,
#27643,#27644,#27645,#27646,#27647,#27648,#27649,#27650,#27651,#27652,#27653,
#27654,#27655,#27656,#27657,#27658,#27659,#27660,#27661,#27662,#27663,#27664,
#27665,#27666,#27667,#27668,#27669,#27670,#27671,#27672,#27673,#27674,#27675,
#27676,#27677,#27678,#27679,#27680,#27681,#27682,#27683,#27684,#27685,#27686,
#27687,#27688,#27689,#27690,#27691,#27692,#27693,#27694,#27695,#27696,#27697,
#27698,#27699,#27700,#27701,#27702,#27703,#27704,#27705,#27706,#27707,#27708,
#27709,#27710,#27711,#27712,#27713,#27714,#27715,#27716,#27717,#27718,#27719));
#29550=AXIS2_PLACEMENT_3D('',#127841,#34129,#34130);
#29551=AXIS2_PLACEMENT_3D('',#127842,#34131,#34132);
#29552=AXIS2_PLACEMENT_3D('',#127844,#34133,#34134);
#29553=AXIS2_PLACEMENT_3D('',#127847,#34136,#34137);
#29554=AXIS2_PLACEMENT_3D('',#127848,#34138,#34139);
#29555=AXIS2_PLACEMENT_3D('',#127851,#34140,#34141);
#29556=AXIS2_PLACEMENT_3D('',#127855,#34143,#34144);
#29557=AXIS2_PLACEMENT_3D('',#127857,#34146,#34147);
#29558=AXIS2_PLACEMENT_3D('',#127863,#34151,#34152);
#29559=AXIS2_PLACEMENT_3D('',#127869,#34156,#34157);
#29560=AXIS2_PLACEMENT_3D('',#127875,#34161,#34162);
#29561=AXIS2_PLACEMENT_3D('',#127881,#34166,#34167);
#29562=AXIS2_PLACEMENT_3D('',#127887,#34171,#34172);
#29563=AXIS2_PLACEMENT_3D('',#127889,#34173,#34174);
#29564=AXIS2_PLACEMENT_3D('',#127891,#34175,#34176);
#29565=AXIS2_PLACEMENT_3D('',#127893,#34178,#34179);
#29566=AXIS2_PLACEMENT_3D('',#127899,#34183,#34184);
#29567=AXIS2_PLACEMENT_3D('',#127905,#34188,#34189);
#29568=AXIS2_PLACEMENT_3D('',#127907,#34190,#34191);
#29569=AXIS2_PLACEMENT_3D('',#127909,#34192,#34193);
#29570=AXIS2_PLACEMENT_3D('',#127911,#34195,#34196);
#29571=AXIS2_PLACEMENT_3D('',#127913,#34197,#34198);
#29572=AXIS2_PLACEMENT_3D('',#127915,#34199,#34200);
#29573=AXIS2_PLACEMENT_3D('',#127917,#34202,#34203);
#29574=AXIS2_PLACEMENT_3D('',#127919,#34204,#34205);
#29575=AXIS2_PLACEMENT_3D('',#127921,#34206,#34207);
#29576=AXIS2_PLACEMENT_3D('',#127923,#34209,#34210);
#29577=AXIS2_PLACEMENT_3D('',#127929,#34214,#34215);
#29578=AXIS2_PLACEMENT_3D('',#127935,#34219,#34220);
#29579=AXIS2_PLACEMENT_3D('',#127941,#34224,#34225);
#29580=AXIS2_PLACEMENT_3D('',#127943,#34226,#34227);
#29581=AXIS2_PLACEMENT_3D('',#127945,#34228,#34229);
#29582=AXIS2_PLACEMENT_3D('',#127947,#34231,#34232);
#29583=AXIS2_PLACEMENT_3D('',#127953,#34236,#34237);
#29584=AXIS2_PLACEMENT_3D('',#127955,#34238,#34239);
#29585=AXIS2_PLACEMENT_3D('',#127957,#34240,#34241);
#29586=AXIS2_PLACEMENT_3D('',#127959,#34243,#34244);
#29587=AXIS2_PLACEMENT_3D('',#127965,#34248,#34249);
#29588=AXIS2_PLACEMENT_3D('',#127967,#34250,#34251);
#29589=AXIS2_PLACEMENT_3D('',#127969,#34252,#34253);
#29590=AXIS2_PLACEMENT_3D('',#127971,#34255,#34256);
#29591=AXIS2_PLACEMENT_3D('',#127977,#34260,#34261);
#29592=AXIS2_PLACEMENT_3D('',#127983,#34265,#34266);
#29593=AXIS2_PLACEMENT_3D('',#127989,#34270,#34271);
#29594=AXIS2_PLACEMENT_3D('',#127991,#34272,#34273);
#29595=AXIS2_PLACEMENT_3D('',#127993,#34274,#34275);
#29596=AXIS2_PLACEMENT_3D('',#127995,#34277,#34278);
#29597=AXIS2_PLACEMENT_3D('',#128001,#34282,#34283);
#29598=AXIS2_PLACEMENT_3D('',#128003,#34284,#34285);
#29599=AXIS2_PLACEMENT_3D('',#128005,#34286,#34287);
#29600=AXIS2_PLACEMENT_3D('',#128007,#34289,#34290);
#29601=AXIS2_PLACEMENT_3D('',#128013,#34294,#34295);
#29602=AXIS2_PLACEMENT_3D('',#128015,#34296,#34297);
#29603=AXIS2_PLACEMENT_3D('',#128017,#34298,#34299);
#29604=AXIS2_PLACEMENT_3D('',#128019,#34301,#34302);
#29605=AXIS2_PLACEMENT_3D('',#128025,#34306,#34307);
#29606=AXIS2_PLACEMENT_3D('',#128027,#34308,#34309);
#29607=AXIS2_PLACEMENT_3D('',#128029,#34310,#34311);
#29608=AXIS2_PLACEMENT_3D('',#128031,#34313,#34314);
#29609=AXIS2_PLACEMENT_3D('',#128037,#34318,#34319);
#29610=AXIS2_PLACEMENT_3D('',#128043,#34323,#34324);
#29611=AXIS2_PLACEMENT_3D('',#128049,#34328,#34329);
#29612=AXIS2_PLACEMENT_3D('',#128051,#34330,#34331);
#29613=AXIS2_PLACEMENT_3D('',#128053,#34332,#34333);
#29614=AXIS2_PLACEMENT_3D('',#128055,#34335,#34336);
#29615=AXIS2_PLACEMENT_3D('',#128061,#34340,#34341);
#29616=AXIS2_PLACEMENT_3D('',#128063,#34342,#34343);
#29617=AXIS2_PLACEMENT_3D('',#128065,#34344,#34345);
#29618=AXIS2_PLACEMENT_3D('',#128067,#34347,#34348);
#29619=AXIS2_PLACEMENT_3D('',#128073,#34352,#34353);
#29620=AXIS2_PLACEMENT_3D('',#128075,#34354,#34355);
#29621=AXIS2_PLACEMENT_3D('',#128077,#34356,#34357);
#29622=AXIS2_PLACEMENT_3D('',#128079,#34359,#34360);
#29623=AXIS2_PLACEMENT_3D('',#128085,#34364,#34365);
#29624=AXIS2_PLACEMENT_3D('',#128091,#34369,#34370);
#29625=AXIS2_PLACEMENT_3D('',#128097,#34374,#34375);
#29626=AXIS2_PLACEMENT_3D('',#128099,#34376,#34377);
#29627=AXIS2_PLACEMENT_3D('',#128101,#34378,#34379);
#29628=AXIS2_PLACEMENT_3D('',#128103,#34381,#34382);
#29629=AXIS2_PLACEMENT_3D('',#128105,#34383,#34384);
#29630=AXIS2_PLACEMENT_3D('',#128107,#34385,#34386);
#29631=AXIS2_PLACEMENT_3D('',#128109,#34388,#34389);
#29632=AXIS2_PLACEMENT_3D('',#128111,#34390,#34391);
#29633=AXIS2_PLACEMENT_3D('',#128113,#34392,#34393);
#29634=AXIS2_PLACEMENT_3D('',#128115,#34395,#34396);
#29635=AXIS2_PLACEMENT_3D('',#128121,#34400,#34401);
#29636=AXIS2_PLACEMENT_3D('',#128127,#34405,#34406);
#29637=AXIS2_PLACEMENT_3D('',#128129,#34407,#34408);
#29638=AXIS2_PLACEMENT_3D('',#128131,#34409,#34410);
#29639=AXIS2_PLACEMENT_3D('',#128133,#34412,#34413);
#29640=AXIS2_PLACEMENT_3D('',#128139,#34417,#34418);
#29641=AXIS2_PLACEMENT_3D('',#128145,#34422,#34423);
#29642=AXIS2_PLACEMENT_3D('',#128151,#34427,#34428);
#29643=AXIS2_PLACEMENT_3D('',#128157,#34432,#34433);
#29644=AXIS2_PLACEMENT_3D('',#128163,#34437,#34438);
#29645=AXIS2_PLACEMENT_3D('',#128165,#34439,#34440);
#29646=AXIS2_PLACEMENT_3D('',#128167,#34441,#34442);
#29647=AXIS2_PLACEMENT_3D('',#128169,#34444,#34445);
#29648=AXIS2_PLACEMENT_3D('',#128175,#34449,#34450);
#29649=AXIS2_PLACEMENT_3D('',#128181,#34454,#34455);
#29650=AXIS2_PLACEMENT_3D('',#128183,#34456,#34457);
#29651=AXIS2_PLACEMENT_3D('',#128185,#34458,#34459);
#29652=AXIS2_PLACEMENT_3D('',#128187,#34461,#34462);
#29653=AXIS2_PLACEMENT_3D('',#128189,#34463,#34464);
#29654=AXIS2_PLACEMENT_3D('',#128191,#34465,#34466);
#29655=AXIS2_PLACEMENT_3D('',#128193,#34468,#34469);
#29656=AXIS2_PLACEMENT_3D('',#128195,#34470,#34471);
#29657=AXIS2_PLACEMENT_3D('',#128197,#34472,#34473);
#29658=AXIS2_PLACEMENT_3D('',#128199,#34475,#34476);
#29659=AXIS2_PLACEMENT_3D('',#128205,#34480,#34481);
#29660=AXIS2_PLACEMENT_3D('',#128211,#34485,#34486);
#29661=AXIS2_PLACEMENT_3D('',#128217,#34490,#34491);
#29662=AXIS2_PLACEMENT_3D('',#128219,#34492,#34493);
#29663=AXIS2_PLACEMENT_3D('',#128221,#34494,#34495);
#29664=AXIS2_PLACEMENT_3D('',#128223,#34497,#34498);
#29665=AXIS2_PLACEMENT_3D('',#128229,#34502,#34503);
#29666=AXIS2_PLACEMENT_3D('',#128231,#34504,#34505);
#29667=AXIS2_PLACEMENT_3D('',#128233,#34506,#34507);
#29668=AXIS2_PLACEMENT_3D('',#128235,#34509,#34510);
#29669=AXIS2_PLACEMENT_3D('',#128241,#34514,#34515);
#29670=AXIS2_PLACEMENT_3D('',#128243,#34516,#34517);
#29671=AXIS2_PLACEMENT_3D('',#128245,#34518,#34519);
#29672=AXIS2_PLACEMENT_3D('',#128247,#34521,#34522);
#29673=AXIS2_PLACEMENT_3D('',#128253,#34526,#34527);
#29674=AXIS2_PLACEMENT_3D('',#128259,#34531,#34532);
#29675=AXIS2_PLACEMENT_3D('',#128265,#34536,#34537);
#29676=AXIS2_PLACEMENT_3D('',#128267,#34538,#34539);
#29677=AXIS2_PLACEMENT_3D('',#128269,#34540,#34541);
#29678=AXIS2_PLACEMENT_3D('',#128271,#34543,#34544);
#29679=AXIS2_PLACEMENT_3D('',#128277,#34548,#34549);
#29680=AXIS2_PLACEMENT_3D('',#128279,#34550,#34551);
#29681=AXIS2_PLACEMENT_3D('',#128281,#34552,#34553);
#29682=AXIS2_PLACEMENT_3D('',#128283,#34555,#34556);
#29683=AXIS2_PLACEMENT_3D('',#128289,#34560,#34561);
#29684=AXIS2_PLACEMENT_3D('',#128291,#34562,#34563);
#29685=AXIS2_PLACEMENT_3D('',#128293,#34564,#34565);
#29686=AXIS2_PLACEMENT_3D('',#128295,#34567,#34568);
#29687=AXIS2_PLACEMENT_3D('',#128301,#34572,#34573);
#29688=AXIS2_PLACEMENT_3D('',#128303,#34574,#34575);
#29689=AXIS2_PLACEMENT_3D('',#128305,#34576,#34577);
#29690=AXIS2_PLACEMENT_3D('',#128307,#34579,#34580);
#29691=AXIS2_PLACEMENT_3D('',#128313,#34584,#34585);
#29692=AXIS2_PLACEMENT_3D('',#128319,#34589,#34590);
#29693=AXIS2_PLACEMENT_3D('',#128325,#34594,#34595);
#29694=AXIS2_PLACEMENT_3D('',#128327,#34596,#34597);
#29695=AXIS2_PLACEMENT_3D('',#128329,#34598,#34599);
#29696=AXIS2_PLACEMENT_3D('',#128331,#34601,#34602);
#29697=AXIS2_PLACEMENT_3D('',#128337,#34606,#34607);
#29698=AXIS2_PLACEMENT_3D('',#128339,#34608,#34609);
#29699=AXIS2_PLACEMENT_3D('',#128341,#34610,#34611);
#29700=AXIS2_PLACEMENT_3D('',#128343,#34613,#34614);
#29701=AXIS2_PLACEMENT_3D('',#128349,#34618,#34619);
#29702=AXIS2_PLACEMENT_3D('',#128351,#34620,#34621);
#29703=AXIS2_PLACEMENT_3D('',#128353,#34622,#34623);
#29704=AXIS2_PLACEMENT_3D('',#128355,#34625,#34626);
#29705=AXIS2_PLACEMENT_3D('',#128361,#34630,#34631);
#29706=AXIS2_PLACEMENT_3D('',#128367,#34635,#34636);
#29707=AXIS2_PLACEMENT_3D('',#128373,#34640,#34641);
#29708=AXIS2_PLACEMENT_3D('',#128375,#34642,#34643);
#29709=AXIS2_PLACEMENT_3D('',#128377,#34644,#34645);
#29710=AXIS2_PLACEMENT_3D('',#128379,#34647,#34648);
#29711=AXIS2_PLACEMENT_3D('',#128381,#34649,#34650);
#29712=AXIS2_PLACEMENT_3D('',#128383,#34651,#34652);
#29713=AXIS2_PLACEMENT_3D('',#128385,#34654,#34655);
#29714=AXIS2_PLACEMENT_3D('',#128387,#34656,#34657);
#29715=AXIS2_PLACEMENT_3D('',#128389,#34658,#34659);
#29716=AXIS2_PLACEMENT_3D('',#128391,#34661,#34662);
#29717=AXIS2_PLACEMENT_3D('',#128397,#34666,#34667);
#29718=AXIS2_PLACEMENT_3D('',#128400,#34670,#34671);
#29719=AXIS2_PLACEMENT_3D('',#128401,#34672,#34673);
#34129=DIRECTION('axis',(0.,0.,1.));
#34130=DIRECTION('refdir',(1.,0.,0.));
#34131=DIRECTION('center_axis',(0.,0.,1.));
#34132=DIRECTION('ref_axis',(1.,0.,0.));
#34133=DIRECTION('center_axis',(0.,0.,-1.));
#34134=DIRECTION('ref_axis',(1.,0.,0.));
#34135=DIRECTION('',(0.,0.,1.));
#34136=DIRECTION('center_axis',(0.,0.,-1.));
#34137=DIRECTION('ref_axis',(1.,0.,0.));
#34138=DIRECTION('center_axis',(0.,0.,1.));
#34139=DIRECTION('ref_axis',(1.76313947997109E-5,-0.999999999844567,0.));
#34140=DIRECTION('center_axis',(0.,0.,1.));
#34141=DIRECTION('ref_axis',(1.76313947997109E-5,-0.999999999844567,0.));
#34142=DIRECTION('',(0.,0.,1.));
#34143=DIRECTION('center_axis',(0.,0.,1.));
#34144=DIRECTION('ref_axis',(1.76313947997109E-5,-0.999999999844567,0.));
#34145=DIRECTION('',(0.,0.,1.));
#34146=DIRECTION('center_axis',(0.000247476788645072,-0.999999969377619,
0.));
#34147=DIRECTION('ref_axis',(0.999999969377619,0.000247476788645072,0.));
#34148=DIRECTION('',(-0.999999969377619,-0.000247476788645072,0.));
#34149=DIRECTION('',(0.999999969377619,0.000247476788645072,0.));
#34150=DIRECTION('',(0.,0.,1.));
#34151=DIRECTION('center_axis',(-0.965913556273921,-0.258864833081411,0.));
#34152=DIRECTION('ref_axis',(0.258864833081411,-0.965913556273921,0.));
#34153=DIRECTION('',(0.258864833081411,-0.965913556273921,0.));
#34154=DIRECTION('',(0.258864833081411,-0.965913556273921,0.));
#34155=DIRECTION('',(0.,0.,1.));
#34156=DIRECTION('center_axis',(0.,-1.,0.));
#34157=DIRECTION('ref_axis',(1.,0.,0.));
#34158=DIRECTION('',(1.,0.,0.));
#34159=DIRECTION('',(1.,0.,0.));
#34160=DIRECTION('',(0.,0.,1.));
#34161=DIRECTION('center_axis',(0.965913556273921,-0.258864833081411,0.));
#34162=DIRECTION('ref_axis',(0.258864833081411,0.965913556273921,0.));
#34163=DIRECTION('',(-0.258864833081411,-0.965913556273921,0.));
#34164=DIRECTION('',(0.258864833081411,0.965913556273921,0.));
#34165=DIRECTION('',(0.,0.,1.));
#34166=DIRECTION('center_axis',(-0.000247476788645237,-0.999999969377619,
0.));
#34167=DIRECTION('ref_axis',(0.999999969377619,-0.000247476788645237,0.));
#34168=DIRECTION('',(0.999999969377619,-0.000247476788645237,0.));
#34169=DIRECTION('',(0.999999969377619,-0.000247476788645237,0.));
#34170=DIRECTION('',(0.,0.,1.));
#34171=DIRECTION('center_axis',(0.,0.,1.));
#34172=DIRECTION('ref_axis',(-0.999999999844567,1.76313947908291E-5,0.));
#34173=DIRECTION('center_axis',(0.,0.,1.));
#34174=DIRECTION('ref_axis',(-0.999999999844567,1.76313947908291E-5,0.));
#34175=DIRECTION('center_axis',(0.,0.,1.));
#34176=DIRECTION('ref_axis',(-0.999999999844567,1.76313947908291E-5,0.));
#34177=DIRECTION('',(0.,0.,1.));
#34178=DIRECTION('center_axis',(-0.999999999844567,1.76313948019314E-5,
0.));
#34179=DIRECTION('ref_axis',(-1.76313948019314E-5,-0.999999999844567,0.));
#34180=DIRECTION('',(1.76313948019314E-5,0.999999999844567,0.));
#34181=DIRECTION('',(-1.76313948019314E-5,-0.999999999844567,0.));
#34182=DIRECTION('',(0.,0.,1.));
#34183=DIRECTION('center_axis',(-0.707094313797817,0.707119248355463,0.));
#34184=DIRECTION('ref_axis',(-0.707119248355463,-0.707094313797817,0.));
#34185=DIRECTION('',(0.707119248355463,0.707094313797817,0.));
#34186=DIRECTION('',(-0.707119248355463,-0.707094313797817,0.));
#34187=DIRECTION('',(0.,0.,1.));
#34188=DIRECTION('center_axis',(0.,0.,1.));
#34189=DIRECTION('ref_axis',(0.586386638808598,0.81003130175738,0.));
#34190=DIRECTION('center_axis',(0.,0.,1.));
#34191=DIRECTION('ref_axis',(0.586386638808598,0.81003130175738,0.));
#34192=DIRECTION('center_axis',(0.,0.,1.));
#34193=DIRECTION('ref_axis',(0.586386638808598,0.81003130175738,0.));
#34194=DIRECTION('',(0.,0.,1.));
#34195=DIRECTION('center_axis',(0.,0.,1.));
#34196=DIRECTION('ref_axis',(0.999993170091859,0.00369591255780612,0.));
#34197=DIRECTION('center_axis',(0.,0.,1.));
#34198=DIRECTION('ref_axis',(-0.586386638808589,-0.810031301757386,0.));
#34199=DIRECTION('center_axis',(0.,0.,-1.));
#34200=DIRECTION('ref_axis',(-0.586386638808589,-0.810031301757386,0.));
#34201=DIRECTION('',(0.,0.,1.));
#34202=DIRECTION('center_axis',(0.,0.,1.));
#34203=DIRECTION('ref_axis',(-0.707119248355468,-0.707094313797812,0.));
#34204=DIRECTION('center_axis',(0.,0.,1.));
#34205=DIRECTION('ref_axis',(-0.707119248355468,-0.707094313797812,0.));
#34206=DIRECTION('center_axis',(0.,0.,1.));
#34207=DIRECTION('ref_axis',(-0.707119248355468,-0.707094313797812,0.));
#34208=DIRECTION('',(0.,0.,1.));
#34209=DIRECTION('center_axis',(-0.707119248355465,-0.707094313797815,0.));
#34210=DIRECTION('ref_axis',(0.707094313797815,-0.707119248355465,0.));
#34211=DIRECTION('',(0.707094313797815,-0.707119248355465,0.));
#34212=DIRECTION('',(0.707094313797815,-0.707119248355465,0.));
#34213=DIRECTION('',(0.,0.,1.));
#34214=DIRECTION('center_axis',(-0.999999999844567,1.76313948004511E-5,
0.));
#34215=DIRECTION('ref_axis',(-1.76313948004511E-5,-0.999999999844567,0.));
#34216=DIRECTION('',(1.76313948004511E-5,0.999999999844567,0.));
#34217=DIRECTION('',(-1.76313948004511E-5,-0.999999999844567,0.));
#34218=DIRECTION('',(0.,0.,1.));
#34219=DIRECTION('center_axis',(-0.707119248355464,-0.707094313797816,0.));
#34220=DIRECTION('ref_axis',(0.707094313797816,-0.707119248355464,0.));
#34221=DIRECTION('',(-0.707094313797816,0.707119248355464,0.));
#34222=DIRECTION('',(0.707094313797816,-0.707119248355464,0.));
#34223=DIRECTION('',(0.,0.,1.));
#34224=DIRECTION('center_axis',(0.,0.,1.));
#34225=DIRECTION('ref_axis',(0.707119248355461,0.707094313797818,0.));
#34226=DIRECTION('center_axis',(0.,0.,1.));
#34227=DIRECTION('ref_axis',(0.707119248355461,0.707094313797818,0.));
#34228=DIRECTION('center_axis',(0.,0.,-1.));
#34229=DIRECTION('ref_axis',(0.707119248355461,0.707094313797818,0.));
#34230=DIRECTION('',(0.,0.,1.));
#34231=DIRECTION('center_axis',(-1.76313948097558E-5,-0.999999999844567,
0.));
#34232=DIRECTION('ref_axis',(0.999999999844567,-1.76313948097558E-5,0.));
#34233=DIRECTION('',(-0.999999999844567,1.76313948097558E-5,0.));
#34234=DIRECTION('',(0.999999999844567,-1.76313948097558E-5,0.));
#34235=DIRECTION('',(0.,0.,1.));
#34236=DIRECTION('center_axis',(0.,0.,1.));
#34237=DIRECTION('ref_axis',(-0.999999999844567,1.76313948019314E-5,0.));
#34238=DIRECTION('center_axis',(0.,0.,1.));
#34239=DIRECTION('ref_axis',(-0.999999999844567,1.76313948019314E-5,0.));
#34240=DIRECTION('center_axis',(0.,0.,1.));
#34241=DIRECTION('ref_axis',(-0.999999999844567,1.76313948019314E-5,0.));
#34242=DIRECTION('',(0.,0.,1.));
#34243=DIRECTION('center_axis',(-0.999999999844567,1.76313947990255E-5,
0.));
#34244=DIRECTION('ref_axis',(-1.76313947990255E-5,-0.999999999844567,0.));
#34245=DIRECTION('',(1.76313947990255E-5,0.999999999844567,0.));
#34246=DIRECTION('',(-1.76313947990255E-5,-0.999999999844567,0.));
#34247=DIRECTION('',(0.,0.,1.));
#34248=DIRECTION('center_axis',(0.,0.,1.));
#34249=DIRECTION('ref_axis',(1.76313947886088E-5,0.999999999844567,0.));
#34250=DIRECTION('center_axis',(0.,0.,1.));
#34251=DIRECTION('ref_axis',(1.76313947886088E-5,0.999999999844567,0.));
#34252=DIRECTION('center_axis',(0.,0.,1.));
#34253=DIRECTION('ref_axis',(1.76313947886088E-5,0.999999999844567,0.));
#34254=DIRECTION('',(0.,0.,1.));
#34255=DIRECTION('center_axis',(1.76313947987393E-5,0.999999999844567,0.));
#34256=DIRECTION('ref_axis',(-0.999999999844567,1.76313947987393E-5,0.));
#34257=DIRECTION('',(0.999999999844567,-1.76313947987393E-5,0.));
#34258=DIRECTION('',(-0.999999999844567,1.76313947987393E-5,0.));
#34259=DIRECTION('',(0.,0.,1.));
#34260=DIRECTION('center_axis',(0.469487130310524,0.882939315283213,0.));
#34261=DIRECTION('ref_axis',(-0.882939315283213,0.469487130310524,0.));
#34262=DIRECTION('',(0.882939315283213,-0.469487130310524,0.));
#34263=DIRECTION('',(-0.882939315283213,0.469487130310524,0.));
#34264=DIRECTION('',(0.,0.,1.));
#34265=DIRECTION('center_axis',(0.999999999844567,-1.76313947965879E-5,
0.));
#34266=DIRECTION('ref_axis',(1.76313947965879E-5,0.999999999844567,0.));
#34267=DIRECTION('',(-1.76313947965879E-5,-0.999999999844567,0.));
#34268=DIRECTION('',(1.76313947965879E-5,0.999999999844567,0.));
#34269=DIRECTION('',(0.,0.,1.));
#34270=DIRECTION('center_axis',(0.,0.,1.));
#34271=DIRECTION('ref_axis',(-0.999999999844567,1.76313947986007E-5,0.));
#34272=DIRECTION('center_axis',(0.,0.,1.));
#34273=DIRECTION('ref_axis',(-0.999999999844567,1.76313947986007E-5,0.));
#34274=DIRECTION('center_axis',(0.,0.,-1.));
#34275=DIRECTION('ref_axis',(-0.999999999844567,1.76313947986007E-5,0.));
#34276=DIRECTION('',(0.,0.,1.));
#34277=DIRECTION('center_axis',(-0.707100547519659,0.707113014798482,0.));
#34278=DIRECTION('ref_axis',(-0.707113014798482,-0.707100547519659,0.));
#34279=DIRECTION('',(0.707113014798482,0.707100547519659,0.));
#34280=DIRECTION('',(-0.707113014798482,-0.707100547519659,0.));
#34281=DIRECTION('',(0.,0.,1.));
#34282=DIRECTION('center_axis',(0.,0.,1.));
#34283=DIRECTION('ref_axis',(0.707100547519658,-0.707113014798483,0.));
#34284=DIRECTION('center_axis',(0.,0.,1.));
#34285=DIRECTION('ref_axis',(0.707100547519658,-0.707113014798483,0.));
#34286=DIRECTION('center_axis',(0.,0.,-1.));
#34287=DIRECTION('ref_axis',(0.707100547519658,-0.707113014798483,0.));
#34288=DIRECTION('',(0.,0.,1.));
#34289=DIRECTION('center_axis',(-0.999999999961142,8.81569739766863E-6,
0.));
#34290=DIRECTION('ref_axis',(-8.81569739766863E-6,-0.999999999961142,0.));
#34291=DIRECTION('',(-8.81569739766863E-6,-0.999999999961142,0.));
#34292=DIRECTION('',(-8.81569739766863E-6,-0.999999999961142,0.));
#34293=DIRECTION('',(0.,0.,1.));
#34294=DIRECTION('center_axis',(0.,0.,1.));
#34295=DIRECTION('ref_axis',(0.999999999961142,-8.8156974001885E-6,0.));
#34296=DIRECTION('center_axis',(0.,0.,1.));
#34297=DIRECTION('ref_axis',(0.999999999961142,-8.8156974001885E-6,0.));
#34298=DIRECTION('center_axis',(0.,0.,-1.));
#34299=DIRECTION('ref_axis',(0.999999999961142,-8.8156974001885E-6,0.));
#34300=DIRECTION('',(0.,0.,1.));
#34301=DIRECTION('center_axis',(-0.707113014798484,-0.707100547519657,0.));
#34302=DIRECTION('ref_axis',(0.707100547519657,-0.707113014798484,0.));
#34303=DIRECTION('',(0.707100547519657,-0.707113014798484,0.));
#34304=DIRECTION('',(0.707100547519657,-0.707113014798484,0.));
#34305=DIRECTION('',(0.,0.,1.));
#34306=DIRECTION('center_axis',(0.,0.,1.));
#34307=DIRECTION('ref_axis',(0.707113014798483,0.707100547519659,0.));
#34308=DIRECTION('center_axis',(0.,0.,1.));
#34309=DIRECTION('ref_axis',(0.707113014798483,0.707100547519659,0.));
#34310=DIRECTION('center_axis',(0.,0.,-1.));
#34311=DIRECTION('ref_axis',(0.707113014798483,0.707100547519659,0.));
#34312=DIRECTION('',(0.,0.,1.));
#34313=DIRECTION('center_axis',(1.,0.,0.));
#34314=DIRECTION('ref_axis',(0.,1.,0.));
#34315=DIRECTION('',(0.,1.,0.));
#34316=DIRECTION('',(0.,1.,0.));
#34317=DIRECTION('',(0.,0.,1.));
#34318=DIRECTION('center_axis',(0.469471562785889,-0.882947592858928,0.));
#34319=DIRECTION('ref_axis',(0.882947592858928,0.469471562785889,0.));
#34320=DIRECTION('',(0.882947592858928,0.469471562785889,0.));
#34321=DIRECTION('',(0.882947592858928,0.469471562785889,0.));
#34322=DIRECTION('',(0.,0.,1.));
#34323=DIRECTION('center_axis',(0.,-1.,0.));
#34324=DIRECTION('ref_axis',(1.,0.,0.));
#34325=DIRECTION('',(1.,0.,0.));
#34326=DIRECTION('',(1.,0.,0.));
#34327=DIRECTION('',(0.,0.,1.));
#34328=DIRECTION('center_axis',(0.,0.,1.));
#34329=DIRECTION('ref_axis',(-1.,0.,0.));
#34330=DIRECTION('center_axis',(0.,0.,1.));
#34331=DIRECTION('ref_axis',(-1.,0.,0.));
#34332=DIRECTION('center_axis',(0.,0.,1.));
#34333=DIRECTION('ref_axis',(-1.,0.,0.));
#34334=DIRECTION('',(0.,0.,1.));
#34335=DIRECTION('center_axis',(-1.,0.,0.));
#34336=DIRECTION('ref_axis',(0.,-1.,0.));
#34337=DIRECTION('',(0.,-1.,0.));
#34338=DIRECTION('',(0.,-1.,0.));
#34339=DIRECTION('',(0.,0.,1.));
#34340=DIRECTION('center_axis',(0.,0.,1.));
#34341=DIRECTION('ref_axis',(0.,1.,0.));
#34342=DIRECTION('center_axis',(0.,0.,1.));
#34343=DIRECTION('ref_axis',(0.,1.,0.));
#34344=DIRECTION('center_axis',(0.,0.,1.));
#34345=DIRECTION('ref_axis',(0.,1.,0.));
#34346=DIRECTION('',(0.,0.,1.));
#34347=DIRECTION('center_axis',(0.,1.,0.));
#34348=DIRECTION('ref_axis',(-1.,0.,0.));
#34349=DIRECTION('',(-1.,0.,0.));
#34350=DIRECTION('',(-1.,0.,0.));
#34351=DIRECTION('',(0.,0.,1.));
#34352=DIRECTION('center_axis',(0.,0.,1.));
#34353=DIRECTION('ref_axis',(0.,-1.,0.));
#34354=DIRECTION('center_axis',(0.,0.,1.));
#34355=DIRECTION('ref_axis',(0.,-1.,0.));
#34356=DIRECTION('center_axis',(0.,0.,-1.));
#34357=DIRECTION('ref_axis',(0.,-1.,0.));
#34358=DIRECTION('',(0.,0.,1.));
#34359=DIRECTION('center_axis',(-0.707106781186547,0.707106781186548,0.));
#34360=DIRECTION('ref_axis',(-0.707106781186548,-0.707106781186547,0.));
#34361=DIRECTION('',(-0.707106781186548,-0.707106781186547,0.));
#34362=DIRECTION('',(-0.707106781186548,-0.707106781186547,0.));
#34363=DIRECTION('',(0.,0.,1.));
#34364=DIRECTION('center_axis',(-1.,0.,0.));
#34365=DIRECTION('ref_axis',(0.,-1.,0.));
#34366=DIRECTION('',(0.,-1.,0.));
#34367=DIRECTION('',(0.,-1.,0.));
#34368=DIRECTION('',(0.,0.,1.));
#34369=DIRECTION('center_axis',(-0.707106781186548,0.707106781186548,0.));
#34370=DIRECTION('ref_axis',(-0.707106781186548,-0.707106781186548,0.));
#34371=DIRECTION('',(0.707106781186547,0.707106781186547,0.));
#34372=DIRECTION('',(-0.707106781186547,-0.707106781186547,0.));
#34373=DIRECTION('',(0.,0.,1.));
#34374=DIRECTION('center_axis',(0.,0.,1.));
#34375=DIRECTION('ref_axis',(0.586372356735787,0.810041640445797,0.));
#34376=DIRECTION('center_axis',(0.,0.,1.));
#34377=DIRECTION('ref_axis',(0.586372356735787,0.810041640445797,0.));
#34378=DIRECTION('center_axis',(0.,0.,1.));
#34379=DIRECTION('ref_axis',(0.586372356735787,0.810041640445797,0.));
#34380=DIRECTION('',(0.,0.,1.));
#34381=DIRECTION('center_axis',(0.,0.,1.));
#34382=DIRECTION('ref_axis',(0.999993104732582,-0.0037135545358805,0.));
#34383=DIRECTION('center_axis',(0.,0.,1.));
#34384=DIRECTION('ref_axis',(-0.592372410147205,-0.805664277287004,0.));
#34385=DIRECTION('center_axis',(0.,0.,-1.));
#34386=DIRECTION('ref_axis',(-0.592372410147205,-0.805664277287004,0.));
#34387=DIRECTION('',(0.,0.,1.));
#34388=DIRECTION('center_axis',(0.,0.,1.));
#34389=DIRECTION('ref_axis',(-0.707106781186548,-0.707106781186548,0.));
#34390=DIRECTION('center_axis',(0.,0.,1.));
#34391=DIRECTION('ref_axis',(-0.707106781186548,-0.707106781186548,0.));
#34392=DIRECTION('center_axis',(0.,0.,1.));
#34393=DIRECTION('ref_axis',(-0.707106781186548,-0.707106781186548,0.));
#34394=DIRECTION('',(0.,0.,1.));
#34395=DIRECTION('center_axis',(-0.707106781186548,-0.707106781186548,0.));
#34396=DIRECTION('ref_axis',(0.707106781186548,-0.707106781186548,0.));
#34397=DIRECTION('',(0.707106781186547,-0.707106781186547,0.));
#34398=DIRECTION('',(0.707106781186547,-0.707106781186547,0.));
#34399=DIRECTION('',(0.,0.,1.));
#34400=DIRECTION('center_axis',(-1.,0.,0.));
#34401=DIRECTION('ref_axis',(0.,-1.,0.));
#34402=DIRECTION('',(0.,-1.,0.));
#34403=DIRECTION('',(0.,-1.,0.));
#34404=DIRECTION('',(0.,0.,1.));
#34405=DIRECTION('center_axis',(0.,0.,1.));
#34406=DIRECTION('ref_axis',(0.,1.,0.));
#34407=DIRECTION('center_axis',(0.,0.,1.));
#34408=DIRECTION('ref_axis',(0.,1.,0.));
#34409=DIRECTION('center_axis',(0.,0.,1.));
#34410=DIRECTION('ref_axis',(0.,1.,0.));
#34411=DIRECTION('',(0.,0.,1.));
#34412=DIRECTION('center_axis',(0.,1.,0.));
#34413=DIRECTION('ref_axis',(-1.,0.,0.));
#34414=DIRECTION('',(-1.,0.,0.));
#34415=DIRECTION('',(-1.,0.,0.));
#34416=DIRECTION('',(0.,0.,1.));
#34417=DIRECTION('center_axis',(1.,0.,0.));
#34418=DIRECTION('ref_axis',(0.,1.,0.));
#34419=DIRECTION('',(0.,1.,0.));
#34420=DIRECTION('',(0.,1.,0.));
#34421=DIRECTION('',(0.,0.,1.));
#34422=DIRECTION('center_axis',(0.,1.,0.));
#34423=DIRECTION('ref_axis',(-1.,0.,0.));
#34424=DIRECTION('',(1.,0.,0.));
#34425=DIRECTION('',(-1.,0.,0.));
#34426=DIRECTION('',(0.,0.,1.));
#34427=DIRECTION('center_axis',(-1.,0.,0.));
#34428=DIRECTION('ref_axis',(0.,-1.,0.));
#34429=DIRECTION('',(0.,1.,0.));
#34430=DIRECTION('',(0.,-1.,0.));
#34431=DIRECTION('',(0.,0.,1.));
#34432=DIRECTION('center_axis',(0.,1.,0.));
#34433=DIRECTION('ref_axis',(-1.,0.,0.));
#34434=DIRECTION('',(1.,0.,0.));
#34435=DIRECTION('',(-1.,0.,0.));
#34436=DIRECTION('',(0.,0.,1.));
#34437=DIRECTION('center_axis',(0.,0.,1.));
#34438=DIRECTION('ref_axis',(1.,8.88178419700124E-15,0.));
#34439=DIRECTION('center_axis',(0.,0.,1.));
#34440=DIRECTION('ref_axis',(1.,8.88178419700124E-15,0.));
#34441=DIRECTION('center_axis',(0.,0.,1.));
#34442=DIRECTION('ref_axis',(1.,8.88178419700124E-15,0.));
#34443=DIRECTION('',(0.,0.,1.));
#34444=DIRECTION('center_axis',(1.,0.,0.));
#34445=DIRECTION('ref_axis',(0.,1.,0.));
#34446=DIRECTION('',(0.,-1.,0.));
#34447=DIRECTION('',(0.,1.,0.));
#34448=DIRECTION('',(0.,0.,1.));
#34449=DIRECTION('center_axis',(0.707106781186548,-0.707106781186548,0.));
#34450=DIRECTION('ref_axis',(0.707106781186548,0.707106781186548,0.));
#34451=DIRECTION('',(-0.707106781186547,-0.707106781186547,0.));
#34452=DIRECTION('',(0.707106781186547,0.707106781186547,0.));
#34453=DIRECTION('',(0.,0.,1.));
#34454=DIRECTION('center_axis',(0.,0.,1.));
#34455=DIRECTION('ref_axis',(-0.586372356735787,-0.810041640445797,0.));
#34456=DIRECTION('center_axis',(0.,0.,1.));
#34457=DIRECTION('ref_axis',(-0.586372356735787,-0.810041640445797,0.));
#34458=DIRECTION('center_axis',(0.,0.,1.));
#34459=DIRECTION('ref_axis',(-0.586372356735787,-0.810041640445797,0.));
#34460=DIRECTION('',(0.,0.,1.));
#34461=DIRECTION('center_axis',(0.,0.,1.));
#34462=DIRECTION('ref_axis',(-0.999993104772333,-0.00371354383159855,0.));
#34463=DIRECTION('center_axis',(0.,0.,1.));
#34464=DIRECTION('ref_axis',(0.586372356735787,0.810041640445797,0.));
#34465=DIRECTION('center_axis',(0.,0.,-1.));
#34466=DIRECTION('ref_axis',(0.586372356735787,0.810041640445797,0.));
#34467=DIRECTION('',(0.,0.,1.));
#34468=DIRECTION('center_axis',(0.,0.,1.));
#34469=DIRECTION('ref_axis',(0.707106781186548,0.707106781186548,0.));
#34470=DIRECTION('center_axis',(0.,0.,1.));
#34471=DIRECTION('ref_axis',(0.707106781186548,0.707106781186548,0.));
#34472=DIRECTION('center_axis',(0.,0.,1.));
#34473=DIRECTION('ref_axis',(0.707106781186548,0.707106781186548,0.));
#34474=DIRECTION('',(0.,0.,1.));
#34475=DIRECTION('center_axis',(0.707106781186548,0.707106781186548,0.));
#34476=DIRECTION('ref_axis',(-0.707106781186548,0.707106781186548,0.));
#34477=DIRECTION('',(-0.707106781186547,0.707106781186547,0.));
#34478=DIRECTION('',(-0.707106781186547,0.707106781186547,0.));
#34479=DIRECTION('',(0.,0.,1.));
#34480=DIRECTION('center_axis',(1.,0.,0.));
#34481=DIRECTION('ref_axis',(0.,1.,0.));
#34482=DIRECTION('',(0.,-1.,0.));
#34483=DIRECTION('',(0.,1.,0.));
#34484=DIRECTION('',(0.,0.,1.));
#34485=DIRECTION('center_axis',(0.707106781186547,0.707106781186548,0.));
#34486=DIRECTION('ref_axis',(-0.707106781186548,0.707106781186547,0.));
#34487=DIRECTION('',(0.707106781186548,-0.707106781186547,0.));
#34488=DIRECTION('',(-0.707106781186548,0.707106781186547,0.));
#34489=DIRECTION('',(0.,0.,1.));
#34490=DIRECTION('center_axis',(0.,0.,1.));
#34491=DIRECTION('ref_axis',(-0.707106781186546,-0.707106781186549,0.));
#34492=DIRECTION('center_axis',(0.,0.,1.));
#34493=DIRECTION('ref_axis',(-0.707106781186546,-0.707106781186549,0.));
#34494=DIRECTION('center_axis',(0.,0.,-1.));
#34495=DIRECTION('ref_axis',(-0.707106781186546,-0.707106781186549,0.));
#34496=DIRECTION('',(0.,0.,1.));
#34497=DIRECTION('center_axis',(0.,1.,0.));
#34498=DIRECTION('ref_axis',(-1.,0.,0.));
#34499=DIRECTION('',(1.,0.,0.));
#34500=DIRECTION('',(-1.,0.,0.));
#34501=DIRECTION('',(0.,0.,1.));
#34502=DIRECTION('center_axis',(0.,0.,1.));
#34503=DIRECTION('ref_axis',(1.,0.,0.));
#34504=DIRECTION('center_axis',(0.,0.,1.));
#34505=DIRECTION('ref_axis',(1.,0.,0.));
#34506=DIRECTION('center_axis',(0.,0.,1.));
#34507=DIRECTION('ref_axis',(1.,0.,0.));
#34508=DIRECTION('',(0.,0.,1.));
#34509=DIRECTION('center_axis',(1.,0.,0.));
#34510=DIRECTION('ref_axis',(0.,1.,0.));
#34511=DIRECTION('',(0.,-1.,0.));
#34512=DIRECTION('',(0.,1.,0.));
#34513=DIRECTION('',(0.,0.,1.));
#34514=DIRECTION('center_axis',(0.,0.,1.));
#34515=DIRECTION('ref_axis',(0.,-1.,0.));
#34516=DIRECTION('center_axis',(0.,0.,1.));
#34517=DIRECTION('ref_axis',(0.,-1.,0.));
#34518=DIRECTION('center_axis',(0.,0.,1.));
#34519=DIRECTION('ref_axis',(0.,-1.,0.));
#34520=DIRECTION('',(0.,0.,1.));
#34521=DIRECTION('center_axis',(0.,-1.,0.));
#34522=DIRECTION('ref_axis',(1.,0.,0.));
#34523=DIRECTION('',(-1.,0.,0.));
#34524=DIRECTION('',(1.,0.,0.));
#34525=DIRECTION('',(0.,0.,1.));
#34526=DIRECTION('center_axis',(-0.469471562785891,-0.882947592858927,0.));
#34527=DIRECTION('ref_axis',(0.882947592858927,-0.469471562785891,0.));
#34528=DIRECTION('',(-0.882947592858927,0.469471562785891,0.));
#34529=DIRECTION('',(0.882947592858927,-0.469471562785891,0.));
#34530=DIRECTION('',(0.,0.,1.));
#34531=DIRECTION('center_axis',(-1.,0.,0.));
#34532=DIRECTION('ref_axis',(0.,-1.,0.));
#34533=DIRECTION('',(0.,1.,0.));
#34534=DIRECTION('',(0.,-1.,0.));
#34535=DIRECTION('',(0.,0.,1.));
#34536=DIRECTION('center_axis',(0.,0.,1.));
#34537=DIRECTION('ref_axis',(1.,0.,0.));
#34538=DIRECTION('center_axis',(0.,0.,1.));
#34539=DIRECTION('ref_axis',(1.,0.,0.));
#34540=DIRECTION('center_axis',(0.,0.,-1.));
#34541=DIRECTION('ref_axis',(1.,0.,0.));
#34542=DIRECTION('',(0.,0.,1.));
#34543=DIRECTION('center_axis',(0.707113014798485,-0.707100547519656,0.));
#34544=DIRECTION('ref_axis',(0.707100547519656,0.707113014798485,0.));
#34545=DIRECTION('',(-0.707100547519656,-0.707113014798485,0.));
#34546=DIRECTION('',(0.707100547519656,0.707113014798485,0.));
#34547=DIRECTION('',(0.,0.,1.));
#34548=DIRECTION('center_axis',(0.,0.,1.));
#34549=DIRECTION('ref_axis',(-0.707113014798483,0.707100547519658,0.));
#34550=DIRECTION('center_axis',(0.,0.,1.));
#34551=DIRECTION('ref_axis',(-0.707113014798483,0.707100547519658,0.));
#34552=DIRECTION('center_axis',(0.,0.,-1.));
#34553=DIRECTION('ref_axis',(-0.707113014798483,0.707100547519658,0.));
#34554=DIRECTION('',(0.,0.,1.));
#34555=DIRECTION('center_axis',(0.999999999961142,8.81569739766863E-6,0.));
#34556=DIRECTION('ref_axis',(-8.81569739766863E-6,0.999999999961142,0.));
#34557=DIRECTION('',(8.81569739766863E-6,-0.999999999961142,0.));
#34558=DIRECTION('',(-8.81569739766863E-6,0.999999999961142,0.));
#34559=DIRECTION('',(0.,0.,1.));
#34560=DIRECTION('center_axis',(0.,0.,1.));
#34561=DIRECTION('ref_axis',(-0.999999999961142,-8.81569739996647E-6,0.));
#34562=DIRECTION('center_axis',(0.,0.,1.));
#34563=DIRECTION('ref_axis',(-0.999999999961142,-8.81569739996647E-6,0.));
#34564=DIRECTION('center_axis',(0.,0.,-1.));
#34565=DIRECTION('ref_axis',(-0.999999999961142,-8.81569739996647E-6,0.));
#34566=DIRECTION('',(0.,0.,1.));
#34567=DIRECTION('center_axis',(0.707100547519659,0.707113014798482,0.));
#34568=DIRECTION('ref_axis',(-0.707113014798482,0.707100547519659,0.));
#34569=DIRECTION('',(-0.707113014798482,0.707100547519659,0.));
#34570=DIRECTION('',(-0.707113014798482,0.707100547519659,0.));
#34571=DIRECTION('',(0.,0.,1.));
#34572=DIRECTION('center_axis',(0.,0.,1.));
#34573=DIRECTION('ref_axis',(-0.707100547519656,-0.707113014798485,0.));
#34574=DIRECTION('center_axis',(0.,0.,1.));
#34575=DIRECTION('ref_axis',(-0.707100547519656,-0.707113014798485,0.));
#34576=DIRECTION('center_axis',(0.,0.,-1.));
#34577=DIRECTION('ref_axis',(-0.707100547519656,-0.707113014798485,0.));
#34578=DIRECTION('',(0.,0.,1.));
#34579=DIRECTION('center_axis',(-0.999999999844567,-1.76313947965879E-5,
0.));
#34580=DIRECTION('ref_axis',(1.76313947965879E-5,-0.999999999844567,0.));
#34581=DIRECTION('',(1.76313947965879E-5,-0.999999999844567,0.));
#34582=DIRECTION('',(1.76313947965879E-5,-0.999999999844567,0.));
#34583=DIRECTION('',(0.,0.,1.));
#34584=DIRECTION('center_axis',(-0.469487130310524,0.882939315283213,0.));
#34585=DIRECTION('ref_axis',(-0.882939315283213,-0.469487130310524,0.));
#34586=DIRECTION('',(-0.882939315283213,-0.469487130310524,0.));
#34587=DIRECTION('',(-0.882939315283213,-0.469487130310524,0.));
#34588=DIRECTION('',(0.,0.,1.));
#34589=DIRECTION('center_axis',(-1.76313947987393E-5,0.999999999844567,
0.));
#34590=DIRECTION('ref_axis',(-0.999999999844567,-1.76313947987393E-5,0.));
#34591=DIRECTION('',(-0.999999999844567,-1.76313947987393E-5,0.));
#34592=DIRECTION('',(-0.999999999844567,-1.76313947987393E-5,0.));
#34593=DIRECTION('',(0.,0.,1.));
#34594=DIRECTION('center_axis',(0.,0.,1.));
#34595=DIRECTION('ref_axis',(0.999999999844567,1.76313947978603E-5,0.));
#34596=DIRECTION('center_axis',(0.,0.,1.));
#34597=DIRECTION('ref_axis',(0.999999999844567,1.76313947978603E-5,0.));
#34598=DIRECTION('center_axis',(0.,0.,1.));
#34599=DIRECTION('ref_axis',(0.999999999844567,1.76313947978603E-5,0.));
#34600=DIRECTION('',(0.,0.,1.));
#34601=DIRECTION('center_axis',(0.999999999844567,1.76313947990255E-5,0.));
#34602=DIRECTION('ref_axis',(-1.76313947990255E-5,0.999999999844567,0.));
#34603=DIRECTION('',(-1.76313947990255E-5,0.999999999844567,0.));
#34604=DIRECTION('',(-1.76313947990255E-5,0.999999999844567,0.));
#34605=DIRECTION('',(0.,0.,1.));
#34606=DIRECTION('center_axis',(0.,0.,1.));
#34607=DIRECTION('ref_axis',(1.76313947974904E-5,-0.999999999844567,0.));
#34608=DIRECTION('center_axis',(0.,0.,1.));
#34609=DIRECTION('ref_axis',(1.76313947974904E-5,-0.999999999844567,0.));
#34610=DIRECTION('center_axis',(0.,0.,1.));
#34611=DIRECTION('ref_axis',(1.76313947974904E-5,-0.999999999844567,0.));
#34612=DIRECTION('',(0.,0.,1.));
#34613=DIRECTION('center_axis',(1.76313948097558E-5,-0.999999999844567,
0.));
#34614=DIRECTION('ref_axis',(0.999999999844567,1.76313948097558E-5,0.));
#34615=DIRECTION('',(0.999999999844567,1.76313948097558E-5,0.));
#34616=DIRECTION('',(0.999999999844567,1.76313948097558E-5,0.));
#34617=DIRECTION('',(0.,0.,1.));
#34618=DIRECTION('center_axis',(0.,0.,1.));
#34619=DIRECTION('ref_axis',(-1.76313947930495E-5,0.999999999844567,0.));
#34620=DIRECTION('center_axis',(0.,0.,1.));
#34621=DIRECTION('ref_axis',(-1.76313947930495E-5,0.999999999844567,0.));
#34622=DIRECTION('center_axis',(0.,0.,-1.));
#34623=DIRECTION('ref_axis',(-1.76313947930495E-5,0.999999999844567,0.));
#34624=DIRECTION('',(0.,0.,1.));
#34625=DIRECTION('center_axis',(0.707119248355464,-0.707094313797816,0.));
#34626=DIRECTION('ref_axis',(0.707094313797816,0.707119248355464,0.));
#34627=DIRECTION('',(0.707094313797816,0.707119248355464,0.));
#34628=DIRECTION('',(0.707094313797816,0.707119248355464,0.));
#34629=DIRECTION('',(0.,0.,1.));
#34630=DIRECTION('center_axis',(0.999999999844567,1.76313948004511E-5,0.));
#34631=DIRECTION('ref_axis',(-1.76313948004511E-5,0.999999999844567,0.));
#34632=DIRECTION('',(-1.76313948004511E-5,0.999999999844567,0.));
#34633=DIRECTION('',(-1.76313948004511E-5,0.999999999844567,0.));
#34634=DIRECTION('',(0.,0.,1.));
#34635=DIRECTION('center_axis',(0.707119248355465,-0.707094313797815,0.));
#34636=DIRECTION('ref_axis',(0.707094313797815,0.707119248355465,0.));
#34637=DIRECTION('',(-0.707094313797815,-0.707119248355465,0.));
#34638=DIRECTION('',(0.707094313797815,0.707119248355465,0.));
#34639=DIRECTION('',(0.,0.,1.));
#34640=DIRECTION('center_axis',(0.,0.,1.));
#34641=DIRECTION('ref_axis',(-0.586358074480661,-0.810051978882424,0.));
#34642=DIRECTION('center_axis',(0.,0.,1.));
#34643=DIRECTION('ref_axis',(-0.586358074480661,-0.810051978882424,0.));
#34644=DIRECTION('center_axis',(0.,0.,1.));
#34645=DIRECTION('ref_axis',(-0.586358074480661,-0.810051978882424,0.));
#34646=DIRECTION('',(0.,0.,1.));
#34647=DIRECTION('center_axis',(0.,0.,1.));
#34648=DIRECTION('ref_axis',(-0.999993170052296,0.00369592326208568,0.));
#34649=DIRECTION('center_axis',(0.,0.,1.));
#34650=DIRECTION('ref_axis',(0.592358205070174,0.805674721513615,0.));
#34651=DIRECTION('center_axis',(0.,0.,-1.));
#34652=DIRECTION('ref_axis',(0.592358205070174,0.805674721513615,0.));
#34653=DIRECTION('',(0.,0.,1.));
#34654=DIRECTION('center_axis',(0.,0.,1.));
#34655=DIRECTION('ref_axis',(0.707094313797827,0.707119248355453,0.));
#34656=DIRECTION('center_axis',(0.,0.,1.));
#34657=DIRECTION('ref_axis',(0.707094313797827,0.707119248355453,0.));
#34658=DIRECTION('center_axis',(0.,0.,1.));
#34659=DIRECTION('ref_axis',(0.707094313797827,0.707119248355453,0.));
#34660=DIRECTION('',(0.,0.,1.));
#34661=DIRECTION('center_axis',(0.707094313797817,0.707119248355463,0.));
#34662=DIRECTION('ref_axis',(-0.707119248355463,0.707094313797817,0.));
#34663=DIRECTION('',(-0.707119248355463,0.707094313797817,0.));
#34664=DIRECTION('',(-0.707119248355463,0.707094313797817,0.));
#34665=DIRECTION('',(0.,0.,1.));
#34666=DIRECTION('center_axis',(0.999999999844567,1.76313948019314E-5,0.));
#34667=DIRECTION('ref_axis',(-1.76313948019314E-5,0.999999999844567,0.));
#34668=DIRECTION('',(-1.76313948019314E-5,0.999999999844567,0.));
#34669=DIRECTION('',(-1.76313948019314E-5,0.999999999844567,0.));
#34670=DIRECTION('center_axis',(0.,0.,1.));
#34671=DIRECTION('ref_axis',(1.,0.,0.));
#34672=DIRECTION('center_axis',(0.,0.,1.));
#34673=DIRECTION('ref_axis',(1.,0.,0.));
#127841=CARTESIAN_POINT('',(0.,0.,0.));
#127842=CARTESIAN_POINT('Origin',(0.,0.,0.));
#127843=CARTESIAN_POINT('',(-12.5,-1.53080849893419E-15,0.));
#127844=CARTESIAN_POINT('Origin',(0.,0.,0.));
#127845=CARTESIAN_POINT('',(-12.5,-1.53080849893419E-15,400.));
#127846=CARTESIAN_POINT('',(-12.5,-1.53080849893419E-15,0.));
#127847=CARTESIAN_POINT('Origin',(0.,0.,400.));
#127848=CARTESIAN_POINT('Origin',(17.4998349855931,-17.0532626526482,0.));
#127849=CARTESIAN_POINT('',(17.4998526169879,-18.0532626524928,0.));
#127850=CARTESIAN_POINT('',(18.4998349854377,-17.0532450212534,0.));
#127851=CARTESIAN_POINT('Origin',(17.4998349855931,-17.0532626526482,0.));
#127852=CARTESIAN_POINT('',(18.4998349854377,-17.0532450212534,400.));
#127853=CARTESIAN_POINT('',(18.4998349854377,-17.0532450212534,0.));
#127854=CARTESIAN_POINT('',(17.4998526169879,-18.0532626524928,400.));
#127855=CARTESIAN_POINT('Origin',(17.4998349855931,-17.0532626526482,400.));
#127856=CARTESIAN_POINT('',(17.4998526169879,-18.0532626524928,0.));
#127857=CARTESIAN_POINT('Origin',(12.5,-18.0545,0.));
#127858=CARTESIAN_POINT('',(12.5,-18.0545,0.));
#127859=CARTESIAN_POINT('',(17.4998526169879,-18.0532626524928,0.));
#127860=CARTESIAN_POINT('',(12.5,-18.0545,400.));
#127861=CARTESIAN_POINT('',(17.4998526169879,-18.0532626524928,400.));
#127862=CARTESIAN_POINT('',(12.5,-18.0545,0.));
#127863=CARTESIAN_POINT('Origin',(12.165,-16.8045,0.));
#127864=CARTESIAN_POINT('',(12.165,-16.8045,0.));
#127865=CARTESIAN_POINT('',(12.165,-16.8045,0.));
#127866=CARTESIAN_POINT('',(12.165,-16.8045,400.));
#127867=CARTESIAN_POINT('',(12.165,-16.8045,400.));
#127868=CARTESIAN_POINT('',(12.165,-16.8045,0.));
#127869=CARTESIAN_POINT('Origin',(-12.165,-16.8045,0.));
#127870=CARTESIAN_POINT('',(-12.165,-16.8045,0.));
#127871=CARTESIAN_POINT('',(-12.165,-16.8045,0.));
#127872=CARTESIAN_POINT('',(-12.165,-16.8045,400.));
#127873=CARTESIAN_POINT('',(-12.165,-16.8045,400.));
#127874=CARTESIAN_POINT('',(-12.165,-16.8045,0.));
#127875=CARTESIAN_POINT('Origin',(-12.5,-18.0545,0.));
#127876=CARTESIAN_POINT('',(-12.5,-18.0545,0.));
#127877=CARTESIAN_POINT('',(-12.165,-16.8045,0.));
#127878=CARTESIAN_POINT('',(-12.5,-18.0545,400.));
#127879=CARTESIAN_POINT('',(-12.165,-16.8045,400.));
#127880=CARTESIAN_POINT('',(-12.5,-18.0545,0.));
#127881=CARTESIAN_POINT('Origin',(-17.4998526949542,-18.0532626524735,0.));
#127882=CARTESIAN_POINT('',(-17.4998526949542,-18.0532626524735,0.));
#127883=CARTESIAN_POINT('',(-17.4998526949542,-18.0532626524735,0.));
#127884=CARTESIAN_POINT('',(-17.4998526949542,-18.0532626524735,400.));
#127885=CARTESIAN_POINT('',(-17.4998526949542,-18.0532626524735,400.));
#127886=CARTESIAN_POINT('',(-17.4998526949542,-18.0532626524735,0.));
#127887=CARTESIAN_POINT('Origin',(-17.4998349855931,-17.0532626526482,0.));
#127888=CARTESIAN_POINT('',(-18.4998349854377,-17.0532450212534,0.));
#127889=CARTESIAN_POINT('Origin',(-17.4998349855931,-17.0532626526482,0.));
#127890=CARTESIAN_POINT('',(-18.4998349854377,-17.0532450212534,400.));
#127891=CARTESIAN_POINT('Origin',(-17.4998349855931,-17.0532626526482,400.));
#127892=CARTESIAN_POINT('',(-18.4998349854377,-17.0532450212534,0.));
#127893=CARTESIAN_POINT('Origin',(-18.4998261697403,-16.5532450213311,0.));
#127894=CARTESIAN_POINT('',(-18.4998261697403,-16.5532450213311,0.));
#127895=CARTESIAN_POINT('',(-18.4998349854377,-17.0532450212534,0.));
#127896=CARTESIAN_POINT('',(-18.4998261697403,-16.5532450213311,400.));
#127897=CARTESIAN_POINT('',(-18.4998349854377,-17.0532450212534,400.));
#127898=CARTESIAN_POINT('',(-18.4998261697403,-16.5532450213311,0.));
#127899=CARTESIAN_POINT('Origin',(-15.6381145716457,-13.6916343333914,0.));
#127900=CARTESIAN_POINT('',(-15.6381145716457,-13.6916343333914,0.));
#127901=CARTESIAN_POINT('',(-18.4998261697403,-16.5532450213311,0.));
#127902=CARTESIAN_POINT('',(-15.6381145716457,-13.6916343333914,400.));
#127903=CARTESIAN_POINT('',(-18.4998261697403,-16.5532450213311,400.));
#127904=CARTESIAN_POINT('',(-15.6381145716457,-13.6916343333914,0.));
#127905=CARTESIAN_POINT('Origin',(-15.4259862775064,-13.903770107898,0.));
#127906=CARTESIAN_POINT('',(-15.2500702858638,-13.6607607173708,0.));
#127907=CARTESIAN_POINT('Origin',(-15.4259862775064,-13.903770107898,0.));
#127908=CARTESIAN_POINT('',(-15.2500702858638,-13.6607607173708,400.));
#127909=CARTESIAN_POINT('Origin',(-15.4259862775064,-13.903770107898,400.));
#127910=CARTESIAN_POINT('',(-15.2500702858638,-13.6607607173708,0.));
#127911=CARTESIAN_POINT('Origin',(-14.8102803067574,-13.0532372410527,0.));
#127912=CARTESIAN_POINT('',(-15.2545491221624,-12.4489809326903,0.));
#127913=CARTESIAN_POINT('Origin',(-14.8102803067574,-13.0532372410527,0.));
#127914=CARTESIAN_POINT('',(-15.2545491221624,-12.4489809326903,400.));
#127915=CARTESIAN_POINT('Origin',(-14.8102803067574,-13.0532372410527,400.));
#127916=CARTESIAN_POINT('',(-15.2545493158391,-12.4489806895913,0.));
#127917=CARTESIAN_POINT('Origin',(-15.4259562865038,-12.2027701081624,0.));
#127918=CARTESIAN_POINT('',(-15.6380920610105,-12.4148984023017,0.));
#127919=CARTESIAN_POINT('Origin',(-15.4259562865038,-12.2027701081624,0.));
#127920=CARTESIAN_POINT('',(-15.6380920610105,-12.4148984023017,400.));
#127921=CARTESIAN_POINT('Origin',(-15.4259562865038,-12.2027701081624,400.));
#127922=CARTESIAN_POINT('',(-15.6380920610105,-12.4148984023017,0.));
#127923=CARTESIAN_POINT('Origin',(-18.4997027489502,-9.55318680420717,0.));
#127924=CARTESIAN_POINT('',(-18.4997027489502,-9.55318680420717,0.));
#127925=CARTESIAN_POINT('',(-18.4997027489502,-9.55318680420717,0.));
#127926=CARTESIAN_POINT('',(-18.4997027489502,-9.55318680420717,400.));
#127927=CARTESIAN_POINT('',(-18.4997027489502,-9.55318680420717,400.));
#127928=CARTESIAN_POINT('',(-18.4997027489502,-9.55318680420717,0.));
#127929=CARTESIAN_POINT('Origin',(-18.4996895254041,-8.80318680432375,0.));
#127930=CARTESIAN_POINT('',(-18.4996895254041,-8.80318680432375,0.));
#127931=CARTESIAN_POINT('',(-18.4997027489502,-9.55318680420717,0.));
#127932=CARTESIAN_POINT('',(-18.4996895254041,-8.80318680432375,400.));
#127933=CARTESIAN_POINT('',(-18.4997027489502,-9.55318680420717,400.));
#127934=CARTESIAN_POINT('',(-18.4996895254041,-8.80318680432375,0.));
#127935=CARTESIAN_POINT('Origin',(-21.4567579457066,-5.84601410770119,0.));
#127936=CARTESIAN_POINT('',(-21.4567579457066,-5.84601410770119,0.));
#127937=CARTESIAN_POINT('',(-18.4996895254041,-8.80318680432375,0.));
#127938=CARTESIAN_POINT('',(-21.4567579457066,-5.84601410770119,400.));
#127939=CARTESIAN_POINT('',(-18.4996895254041,-8.80318680432375,400.));
#127940=CARTESIAN_POINT('',(-21.4567579457066,-5.84601410770119,0.));
#127941=CARTESIAN_POINT('Origin',(-22.1638771940621,-6.55310842149901,0.));
#127942=CARTESIAN_POINT('',(-22.1638595626673,-5.55310842165444,0.));
#127943=CARTESIAN_POINT('Origin',(-22.1638771940621,-6.55310842149901,0.));
#127944=CARTESIAN_POINT('',(-22.1638595626673,-5.55310842165444,400.));
#127945=CARTESIAN_POINT('Origin',(-22.1638771940621,-6.55310842149901,400.));
#127946=CARTESIAN_POINT('',(-22.1638595626673,-5.55310842165444,0.));
#127947=CARTESIAN_POINT('Origin',(-22.499859562615,-5.55310249750579,0.));
#127948=CARTESIAN_POINT('',(-22.4998595626151,-5.55310249750579,0.));
#127949=CARTESIAN_POINT('',(-22.1638595626673,-5.55310842165444,0.));
#127950=CARTESIAN_POINT('',(-22.4998595626151,-5.55310249750579,400.));
#127951=CARTESIAN_POINT('',(-22.1638595626673,-5.55310842165444,400.));
#127952=CARTESIAN_POINT('',(-22.4998595626151,-5.55310249750579,0.));
#127953=CARTESIAN_POINT('Origin',(-22.4998507469176,-5.0531024975835,0.));
#127954=CARTESIAN_POINT('',(-22.9998507468399,-5.0530936818861,0.));
#127955=CARTESIAN_POINT('Origin',(-22.4998507469176,-5.0531024975835,0.));
#127956=CARTESIAN_POINT('',(-22.9998507468399,-5.0530936818861,400.));
#127957=CARTESIAN_POINT('Origin',(-22.4998507469176,-5.0531024975835,400.));
#127958=CARTESIAN_POINT('',(-22.9998507468399,-5.0530936818861,0.));
#127959=CARTESIAN_POINT('Origin',(-22.999779339691,-1.00309368251561,0.));
#127960=CARTESIAN_POINT('',(-22.999779339691,-1.00309368251561,0.));
#127961=CARTESIAN_POINT('',(-22.9998507468399,-5.0530936818861,0.));
#127962=CARTESIAN_POINT('',(-22.999779339691,-1.00309368251561,400.));
#127963=CARTESIAN_POINT('',(-22.9998507468399,-5.0530936818861,400.));
#127964=CARTESIAN_POINT('',(-22.999779339691,-1.00309368251561,0.));
#127965=CARTESIAN_POINT('Origin',(-22.6997793397376,-1.00309897193405,0.));
#127966=CARTESIAN_POINT('',(-22.6997740503192,-0.703098971980677,0.));
#127967=CARTESIAN_POINT('Origin',(-22.6997793397376,-1.00309897193405,0.));
#127968=CARTESIAN_POINT('',(-22.6997740503192,-0.703098971980677,400.));
#127969=CARTESIAN_POINT('Origin',(-22.6997793397376,-1.00309897193405,400.));
#127970=CARTESIAN_POINT('',(-22.6997740503192,-0.703098971980677,0.));
#127971=CARTESIAN_POINT('Origin',(-21.6997740504746,-0.703116603375476,
0.));
#127972=CARTESIAN_POINT('',(-21.6997740504746,-0.703116603375476,0.));
#127973=CARTESIAN_POINT('',(-22.6997740503192,-0.703098971980677,0.));
#127974=CARTESIAN_POINT('',(-21.6997740504746,-0.703116603375476,400.));
#127975=CARTESIAN_POINT('',(-22.6997740503192,-0.703098971980677,400.));
#127976=CARTESIAN_POINT('',(-21.6997740504746,-0.703116603375476,0.));
#127977=CARTESIAN_POINT('Origin',(-20.999603173455,-1.07541989771172,0.));
#127978=CARTESIAN_POINT('',(-20.999603173455,-1.07541989771172,0.));
#127979=CARTESIAN_POINT('',(-21.6997740504746,-0.703116603375476,0.));
#127980=CARTESIAN_POINT('',(-20.999603173455,-1.07541989771172,400.));
#127981=CARTESIAN_POINT('',(-21.6997740504746,-0.703116603375476,400.));
#127982=CARTESIAN_POINT('',(-20.999603173455,-1.07541989771172,0.));
#127983=CARTESIAN_POINT('Origin',(-20.9996316305262,-2.68941989746085,0.));
#127984=CARTESIAN_POINT('',(-20.9996316305262,-2.68941989746085,0.));
#127985=CARTESIAN_POINT('',(-20.999603173455,-1.07541989771172,0.));
#127986=CARTESIAN_POINT('',(-20.9996316305262,-2.68941989746085,400.));
#127987=CARTESIAN_POINT('',(-20.999603173455,-1.07541989771172,400.));
#127988=CARTESIAN_POINT('',(-20.9996316305262,-2.68941989746085,0.));
#127989=CARTESIAN_POINT('Origin',(-19.9996316306817,-2.68943752885565,0.));
#127990=CARTESIAN_POINT('',(-19.292531083162,-3.39655054365413,0.));
#127991=CARTESIAN_POINT('Origin',(-19.9996316306817,-2.68943752885565,0.));
#127992=CARTESIAN_POINT('',(-19.292531083162,-3.39655054365413,400.));
#127993=CARTESIAN_POINT('Origin',(-19.9996316306817,-2.68943752885565,400.));
#127994=CARTESIAN_POINT('',(-19.292531083162,-3.39655054365413,0.));
#127995=CARTESIAN_POINT('Origin',(-17.9143678173198,-2.01841157653832,0.));
#127996=CARTESIAN_POINT('',(-17.9143678173198,-2.01841157653832,0.));
#127997=CARTESIAN_POINT('',(-19.292531083162,-3.39655054365413,0.));
#127998=CARTESIAN_POINT('',(-17.9143678173198,-2.01841157653832,400.));
#127999=CARTESIAN_POINT('',(-19.292531083162,-3.39655054365413,400.));
#128000=CARTESIAN_POINT('',(-17.9143678173198,-2.01841157653832,0.));
#128001=CARTESIAN_POINT('Origin',(-21.4498705549181,1.5171534974541,0.));
#128002=CARTESIAN_POINT('',(-16.4498705551123,1.5171094189671,0.));
#128003=CARTESIAN_POINT('Origin',(-21.4498705549181,1.5171534974541,0.));
#128004=CARTESIAN_POINT('',(-16.4498705551123,1.5171094189671,400.));
#128005=CARTESIAN_POINT('Origin',(-21.4498705549181,1.5171534974541,400.));
#128006=CARTESIAN_POINT('',(-16.4498705551123,1.5171094189671,0.));
#128007=CARTESIAN_POINT('Origin',(-16.449862991244,2.37510941893376,0.));
#128008=CARTESIAN_POINT('',(-16.449862991244,2.37510941893376,0.));
#128009=CARTESIAN_POINT('',(-16.449862991244,2.37510941893376,0.));
#128010=CARTESIAN_POINT('',(-16.449862991244,2.37510941893376,400.));
#128011=CARTESIAN_POINT('',(-16.449862991244,2.37510941893376,400.));
#128012=CARTESIAN_POINT('',(-16.449862991244,2.37510941893376,0.));
#128013=CARTESIAN_POINT('Origin',(-21.4498629910497,2.37515349742076,0.));
#128014=CARTESIAN_POINT('',(-17.9142979170573,5.91065623501905,0.));
#128015=CARTESIAN_POINT('Origin',(-21.4498629910497,2.37515349742076,0.));
#128016=CARTESIAN_POINT('',(-17.9142979170573,5.91065623501905,400.));
#128017=CARTESIAN_POINT('Origin',(-21.4498629910497,2.37515349742076,400.));
#128018=CARTESIAN_POINT('',(-17.9142979170573,5.91065623501905,0.));
#128019=CARTESIAN_POINT('Origin',(-19.2924368841731,7.28881950086129,0.));
#128020=CARTESIAN_POINT('',(-19.2924368841731,7.28881950086129,0.));
#128021=CARTESIAN_POINT('',(-19.2924368841731,7.28881950086129,0.));
#128022=CARTESIAN_POINT('',(-19.2924368841731,7.28881950086129,400.));
#128023=CARTESIAN_POINT('',(-19.2924368841731,7.28881950086129,400.));
#128024=CARTESIAN_POINT('',(-19.2924368841731,7.28881950086129,0.));
#128025=CARTESIAN_POINT('Origin',(-19.9995498989716,6.58171895334164,0.));
#128026=CARTESIAN_POINT('',(-20.9995498989716,6.58171895334164,0.));
#128027=CARTESIAN_POINT('Origin',(-19.9995498989716,6.58171895334164,0.));
#128028=CARTESIAN_POINT('',(-20.9995498989716,6.58171895334164,400.));
#128029=CARTESIAN_POINT('Origin',(-19.9995498989716,6.58171895334164,400.));
#128030=CARTESIAN_POINT('',(-20.9995498989716,6.58171895334164,0.));
#128031=CARTESIAN_POINT('Origin',(-20.9995498989716,4.96771895334164,0.));
#128032=CARTESIAN_POINT('',(-20.9995498989716,4.96771895334164,0.));
#128033=CARTESIAN_POINT('',(-20.9995498989716,4.96771895334164,0.));
#128034=CARTESIAN_POINT('',(-20.9995498989716,4.96771895334164,400.));
#128035=CARTESIAN_POINT('',(-20.9995498989716,4.96771895334164,400.));
#128036=CARTESIAN_POINT('',(-20.9995498989716,4.96771895334164,0.));
#128037=CARTESIAN_POINT('Origin',(-21.6997273401087,4.59542800405243,0.));
#128038=CARTESIAN_POINT('',(-21.6997273401087,4.59542800405243,0.));
#128039=CARTESIAN_POINT('',(-21.6997273401087,4.59542800405243,0.));
#128040=CARTESIAN_POINT('',(-21.6997273401087,4.59542800405243,400.));
#128041=CARTESIAN_POINT('',(-21.6997273401087,4.59542800405243,400.));
#128042=CARTESIAN_POINT('',(-21.6997273401087,4.59542800405243,0.));
#128043=CARTESIAN_POINT('Origin',(-22.6997273401087,4.59542800405243,0.));
#128044=CARTESIAN_POINT('',(-22.6997273401087,4.59542800405243,0.));
#128045=CARTESIAN_POINT('',(-22.6997273401087,4.59542800405243,0.));
#128046=CARTESIAN_POINT('',(-22.6997273401087,4.59542800405243,400.));
#128047=CARTESIAN_POINT('',(-22.6997273401087,4.59542800405243,400.));
#128048=CARTESIAN_POINT('',(-22.6997273401087,4.59542800405243,0.));
#128049=CARTESIAN_POINT('Origin',(-22.6997273401087,4.89542800405243,0.));
#128050=CARTESIAN_POINT('',(-22.9997273401087,4.89542800405243,0.));
#128051=CARTESIAN_POINT('Origin',(-22.6997273401087,4.89542800405243,0.));
#128052=CARTESIAN_POINT('',(-22.9997273401087,4.89542800405243,400.));
#128053=CARTESIAN_POINT('Origin',(-22.6997273401087,4.89542800405243,400.));
#128054=CARTESIAN_POINT('',(-22.9997273401087,4.89542800405243,0.));
#128055=CARTESIAN_POINT('Origin',(-22.9997273401087,8.94542800405243,0.));
#128056=CARTESIAN_POINT('',(-22.9997273401087,8.94542800405243,0.));
#128057=CARTESIAN_POINT('',(-22.9997273401087,8.94542800405243,0.));
#128058=CARTESIAN_POINT('',(-22.9997273401087,8.94542800405243,400.));
#128059=CARTESIAN_POINT('',(-22.9997273401087,8.94542800405243,400.));
#128060=CARTESIAN_POINT('',(-22.9997273401087,8.94542800405243,0.));
#128061=CARTESIAN_POINT('Origin',(-22.4997273401087,8.94542800405243,0.));
#128062=CARTESIAN_POINT('',(-22.4997273401087,9.44542800405243,0.));
#128063=CARTESIAN_POINT('Origin',(-22.4997273401087,8.94542800405243,0.));
#128064=CARTESIAN_POINT('',(-22.4997273401087,9.44542800405243,400.));
#128065=CARTESIAN_POINT('Origin',(-22.4997273401087,8.94542800405243,400.));
#128066=CARTESIAN_POINT('',(-22.4997273401087,9.44542800405243,0.));
#128067=CARTESIAN_POINT('Origin',(-22.1637273401087,9.44542800405243,0.));
#128068=CARTESIAN_POINT('',(-22.1637273401087,9.44542800405243,0.));
#128069=CARTESIAN_POINT('',(-22.1637273401087,9.44542800405243,0.));
#128070=CARTESIAN_POINT('',(-22.1637273401087,9.44542800405243,400.));
#128071=CARTESIAN_POINT('',(-22.1637273401087,9.44542800405243,400.));
#128072=CARTESIAN_POINT('',(-22.1637273401087,9.44542800405243,0.));
#128073=CARTESIAN_POINT('Origin',(-22.1637273401087,10.4454280040524,0.));
#128074=CARTESIAN_POINT('',(-21.4566205589221,9.73832122286588,0.));
#128075=CARTESIAN_POINT('Origin',(-22.1637273401087,10.4454280040524,0.));
#128076=CARTESIAN_POINT('',(-21.4566205589221,9.73832122286588,400.));
#128077=CARTESIAN_POINT('Origin',(-22.1637273401087,10.4454280040524,400.));
#128078=CARTESIAN_POINT('',(-21.4566205589221,9.73832122286588,0.));
#128079=CARTESIAN_POINT('Origin',(-18.4995,12.695441781788,0.));
#128080=CARTESIAN_POINT('',(-18.4995,12.695441781788,0.));
#128081=CARTESIAN_POINT('',(-18.4995,12.695441781788,0.));
#128082=CARTESIAN_POINT('',(-18.4995,12.695441781788,400.));
#128083=CARTESIAN_POINT('',(-18.4995,12.695441781788,400.));
#128084=CARTESIAN_POINT('',(-18.4995,12.695441781788,0.));
#128085=CARTESIAN_POINT('Origin',(-18.4995,13.445441781788,0.));
#128086=CARTESIAN_POINT('',(-18.4995,13.445441781788,0.));
#128087=CARTESIAN_POINT('',(-18.4995,13.445441781788,0.));
#128088=CARTESIAN_POINT('',(-18.4995,13.445441781788,400.));
#128089=CARTESIAN_POINT('',(-18.4995,13.445441781788,400.));
#128090=CARTESIAN_POINT('',(-18.4995,13.445441781788,0.));
#128091=CARTESIAN_POINT('Origin',(-15.637838856538,16.30710292525,0.));
#128092=CARTESIAN_POINT('',(-15.637838856538,16.30710292525,0.));
#128093=CARTESIAN_POINT('',(-18.4995,13.445441781788,0.));
#128094=CARTESIAN_POINT('',(-15.637838856538,16.30710292525,400.));
#128095=CARTESIAN_POINT('',(-18.4995,13.445441781788,400.));
#128096=CARTESIAN_POINT('',(-15.637838856538,16.30710292525,0.));
#128097=CARTESIAN_POINT('Origin',(-15.4257068221821,16.094970890894,0.));
#128098=CARTESIAN_POINT('',(-15.2542955236899,16.341178459318,0.));
#128099=CARTESIAN_POINT('Origin',(-15.4257068221821,16.094970890894,0.));
#128100=CARTESIAN_POINT('',(-15.2542955236899,16.341178459318,400.));
#128101=CARTESIAN_POINT('Origin',(-15.4257068221821,16.094970890894,400.));
#128102=CARTESIAN_POINT('',(-15.2542955236899,16.341178459318,0.));
#128103=CARTESIAN_POINT('Origin',(-14.8100158476095,16.9454271684259,0.));
#128104=CARTESIAN_POINT('',(-15.2497952977804,17.5529586510386,0.));
#128105=CARTESIAN_POINT('Origin',(-14.8100158476095,16.9454271684259,0.));
#128106=CARTESIAN_POINT('',(-15.2497952977804,17.5529586510386,400.));
#128107=CARTESIAN_POINT('Origin',(-14.8100158476095,16.9454271684259,400.));
#128108=CARTESIAN_POINT('',(-15.2497954798992,17.5529589026258,0.));
#128109=CARTESIAN_POINT('Origin',(-15.4257068221821,17.795970890894,0.));
#128110=CARTESIAN_POINT('',(-15.637838856538,17.583838856538,0.));
#128111=CARTESIAN_POINT('Origin',(-15.4257068221821,17.795970890894,0.));
#128112=CARTESIAN_POINT('',(-15.637838856538,17.583838856538,400.));
#128113=CARTESIAN_POINT('Origin',(-15.4257068221821,17.795970890894,400.));
#128114=CARTESIAN_POINT('',(-15.637838856538,17.583838856538,0.));
#128115=CARTESIAN_POINT('Origin',(-18.4995,20.4455,0.));
#128116=CARTESIAN_POINT('',(-18.4995,20.4455,0.));
#128117=CARTESIAN_POINT('',(-18.4995,20.4455,0.));
#128118=CARTESIAN_POINT('',(-18.4995,20.4455,400.));
#128119=CARTESIAN_POINT('',(-18.4995,20.4455,400.));
#128120=CARTESIAN_POINT('',(-18.4995,20.4455,0.));
#128121=CARTESIAN_POINT('Origin',(-18.4995,20.9455,0.));
#128122=CARTESIAN_POINT('',(-18.4995,20.9455,0.));
#128123=CARTESIAN_POINT('',(-18.4995,20.9455,0.));
#128124=CARTESIAN_POINT('',(-18.4995,20.9455,400.));
#128125=CARTESIAN_POINT('',(-18.4995,20.9455,400.));
#128126=CARTESIAN_POINT('',(-18.4995,20.9455,0.));
#128127=CARTESIAN_POINT('Origin',(-17.4995,20.9455,0.));
#128128=CARTESIAN_POINT('',(-17.4995,21.9455,0.));
#128129=CARTESIAN_POINT('Origin',(-17.4995,20.9455,0.));
#128130=CARTESIAN_POINT('',(-17.4995,21.9455,400.));
#128131=CARTESIAN_POINT('Origin',(-17.4995,20.9455,400.));
#128132=CARTESIAN_POINT('',(-17.4995,21.9455,0.));
#128133=CARTESIAN_POINT('Origin',(-7.0995,21.9455,0.));
#128134=CARTESIAN_POINT('',(-7.0995,21.9455,0.));
#128135=CARTESIAN_POINT('',(-7.0995,21.9455,0.));
#128136=CARTESIAN_POINT('',(-7.0995,21.9455,400.));
#128137=CARTESIAN_POINT('',(-7.0995,21.9455,400.));
#128138=CARTESIAN_POINT('',(-7.0995,21.9455,0.));
#128139=CARTESIAN_POINT('Origin',(-7.0995,16.8045,0.));
#128140=CARTESIAN_POINT('',(-7.0995,16.8045,0.));
#128141=CARTESIAN_POINT('',(-7.0995,16.8045,0.));
#128142=CARTESIAN_POINT('',(-7.0995,16.8045,400.));
#128143=CARTESIAN_POINT('',(-7.0995,16.8045,400.));
#128144=CARTESIAN_POINT('',(-7.0995,16.8045,0.));
#128145=CARTESIAN_POINT('Origin',(7.0995,16.8045,0.));
#128146=CARTESIAN_POINT('',(7.0995,16.8045,0.));
#128147=CARTESIAN_POINT('',(-7.0995,16.8045,0.));
#128148=CARTESIAN_POINT('',(7.0995,16.8045,400.));
#128149=CARTESIAN_POINT('',(-7.0995,16.8045,400.));
#128150=CARTESIAN_POINT('',(7.0995,16.8045,0.));
#128151=CARTESIAN_POINT('Origin',(7.0995,21.9455,0.));
#128152=CARTESIAN_POINT('',(7.0995,21.9455,0.));
#128153=CARTESIAN_POINT('',(7.0995,16.8045,0.));
#128154=CARTESIAN_POINT('',(7.0995,21.9455,400.));
#128155=CARTESIAN_POINT('',(7.0995,16.8045,400.));
#128156=CARTESIAN_POINT('',(7.0995,21.9455,0.));
#128157=CARTESIAN_POINT('Origin',(17.4995,21.9455,0.));
#128158=CARTESIAN_POINT('',(17.4995,21.9455,0.));
#128159=CARTESIAN_POINT('',(7.0995,21.9455,0.));
#128160=CARTESIAN_POINT('',(17.4995,21.9455,400.));
#128161=CARTESIAN_POINT('',(7.0995,21.9455,400.));
#128162=CARTESIAN_POINT('',(17.4995,21.9455,0.));
#128163=CARTESIAN_POINT('Origin',(17.4995,20.9455,0.));
#128164=CARTESIAN_POINT('',(18.4995,20.9455,0.));
#128165=CARTESIAN_POINT('Origin',(17.4995,20.9455,0.));
#128166=CARTESIAN_POINT('',(18.4995,20.9455,400.));
#128167=CARTESIAN_POINT('Origin',(17.4995,20.9455,400.));
#128168=CARTESIAN_POINT('',(18.4995,20.9455,0.));
#128169=CARTESIAN_POINT('Origin',(18.4995,20.4455,0.));
#128170=CARTESIAN_POINT('',(18.4995,20.4455,0.));
#128171=CARTESIAN_POINT('',(18.4995,20.9455,0.));
#128172=CARTESIAN_POINT('',(18.4995,20.4455,400.));
#128173=CARTESIAN_POINT('',(18.4995,20.9455,400.));
#128174=CARTESIAN_POINT('',(18.4995,20.4455,0.));
#128175=CARTESIAN_POINT('Origin',(15.637838856538,17.583838856538,0.));
#128176=CARTESIAN_POINT('',(15.637838856538,17.583838856538,0.));
#128177=CARTESIAN_POINT('',(18.4995,20.4455,0.));
#128178=CARTESIAN_POINT('',(15.637838856538,17.583838856538,400.));
#128179=CARTESIAN_POINT('',(18.4995,20.4455,400.));
#128180=CARTESIAN_POINT('',(15.637838856538,17.583838856538,0.));
#128181=CARTESIAN_POINT('Origin',(15.4257068221821,17.795970890894,0.));
#128182=CARTESIAN_POINT('',(15.2497951151613,17.5529583987603,0.));
#128183=CARTESIAN_POINT('Origin',(15.4257068221821,17.795970890894,0.));
#128184=CARTESIAN_POINT('',(15.2497951151613,17.5529583987603,400.));
#128185=CARTESIAN_POINT('Origin',(15.4257068221821,17.795970890894,400.));
#128186=CARTESIAN_POINT('',(15.2497951151613,17.5529583987603,0.));
#128187=CARTESIAN_POINT('Origin',(14.8100158476095,16.9454271684259,0.));
#128188=CARTESIAN_POINT('',(15.254295316827,16.3411786932362,0.));
#128189=CARTESIAN_POINT('Origin',(14.8100158476095,16.9454271684259,0.));
#128190=CARTESIAN_POINT('',(15.254295316827,16.3411786932362,400.));
#128191=CARTESIAN_POINT('Origin',(14.8100158476095,16.9454271684259,400.));
#128192=CARTESIAN_POINT('',(15.254295510508,16.3411784501406,0.));
#128193=CARTESIAN_POINT('Origin',(15.4257068221821,16.094970890894,0.));
#128194=CARTESIAN_POINT('',(15.637838856538,16.30710292525,0.));
#128195=CARTESIAN_POINT('Origin',(15.4257068221821,16.094970890894,0.));
#128196=CARTESIAN_POINT('',(15.637838856538,16.30710292525,400.));
#128197=CARTESIAN_POINT('Origin',(15.4257068221821,16.094970890894,400.));
#128198=CARTESIAN_POINT('',(15.637838856538,16.30710292525,0.));
#128199=CARTESIAN_POINT('Origin',(18.4995,13.445441781788,0.));
#128200=CARTESIAN_POINT('',(18.4995,13.445441781788,0.));
#128201=CARTESIAN_POINT('',(18.4995,13.445441781788,0.));
#128202=CARTESIAN_POINT('',(18.4995,13.445441781788,400.));
#128203=CARTESIAN_POINT('',(18.4995,13.445441781788,400.));
#128204=CARTESIAN_POINT('',(18.4995,13.445441781788,0.));
#128205=CARTESIAN_POINT('Origin',(18.4995,12.695441781788,0.));
#128206=CARTESIAN_POINT('',(18.4995,12.695441781788,0.));
#128207=CARTESIAN_POINT('',(18.4995,13.445441781788,0.));
#128208=CARTESIAN_POINT('',(18.4995,12.695441781788,400.));
#128209=CARTESIAN_POINT('',(18.4995,13.445441781788,400.));
#128210=CARTESIAN_POINT('',(18.4995,12.695441781788,0.));
#128211=CARTESIAN_POINT('Origin',(21.4566205589221,9.73832122286588,0.));
#128212=CARTESIAN_POINT('',(21.4566205589221,9.73832122286588,0.));
#128213=CARTESIAN_POINT('',(18.4995,12.695441781788,0.));
#128214=CARTESIAN_POINT('',(21.4566205589221,9.73832122286588,400.));
#128215=CARTESIAN_POINT('',(18.4995,12.695441781788,400.));
#128216=CARTESIAN_POINT('',(21.4566205589221,9.73832122286588,0.));
#128217=CARTESIAN_POINT('Origin',(22.1637273401087,10.4454280040524,0.));
#128218=CARTESIAN_POINT('',(22.1637273401087,9.44542800405243,0.));
#128219=CARTESIAN_POINT('Origin',(22.1637273401087,10.4454280040524,0.));
#128220=CARTESIAN_POINT('',(22.1637273401087,9.44542800405243,400.));
#128221=CARTESIAN_POINT('Origin',(22.1637273401087,10.4454280040524,400.));
#128222=CARTESIAN_POINT('',(22.1637273401087,9.44542800405243,0.));
#128223=CARTESIAN_POINT('Origin',(22.4997273401087,9.44542800405243,0.));
#128224=CARTESIAN_POINT('',(22.4997273401087,9.44542800405243,0.));
#128225=CARTESIAN_POINT('',(22.1637273401087,9.44542800405243,0.));
#128226=CARTESIAN_POINT('',(22.4997273401087,9.44542800405243,400.));
#128227=CARTESIAN_POINT('',(22.1637273401087,9.44542800405243,400.));
#128228=CARTESIAN_POINT('',(22.4997273401087,9.44542800405243,0.));
#128229=CARTESIAN_POINT('Origin',(22.4997273401087,8.94542800405243,0.));
#128230=CARTESIAN_POINT('',(22.9997273401087,8.94542800405243,0.));
#128231=CARTESIAN_POINT('Origin',(22.4997273401087,8.94542800405243,0.));
#128232=CARTESIAN_POINT('',(22.9997273401087,8.94542800405243,400.));
#128233=CARTESIAN_POINT('Origin',(22.4997273401087,8.94542800405243,400.));
#128234=CARTESIAN_POINT('',(22.9997273401087,8.94542800405243,0.));
#128235=CARTESIAN_POINT('Origin',(22.9997273401087,4.89542800405242,0.));
#128236=CARTESIAN_POINT('',(22.9997273401087,4.89542800405242,0.));
#128237=CARTESIAN_POINT('',(22.9997273401087,8.94542800405243,0.));
#128238=CARTESIAN_POINT('',(22.9997273401087,4.89542800405242,400.));
#128239=CARTESIAN_POINT('',(22.9997273401087,8.94542800405243,400.));
#128240=CARTESIAN_POINT('',(22.9997273401087,4.89542800405242,0.));
#128241=CARTESIAN_POINT('Origin',(22.6997273401087,4.89542800405242,0.));
#128242=CARTESIAN_POINT('',(22.6997273401087,4.59542800405243,0.));
#128243=CARTESIAN_POINT('Origin',(22.6997273401087,4.89542800405242,0.));
#128244=CARTESIAN_POINT('',(22.6997273401087,4.59542800405243,400.));
#128245=CARTESIAN_POINT('Origin',(22.6997273401087,4.89542800405242,400.));
#128246=CARTESIAN_POINT('',(22.6997273401087,4.59542800405243,0.));
#128247=CARTESIAN_POINT('Origin',(21.6997273401087,4.59542800405243,0.));
#128248=CARTESIAN_POINT('',(21.6997273401087,4.59542800405243,0.));
#128249=CARTESIAN_POINT('',(22.6997273401087,4.59542800405243,0.));
#128250=CARTESIAN_POINT('',(21.6997273401087,4.59542800405243,400.));
#128251=CARTESIAN_POINT('',(22.6997273401087,4.59542800405243,400.));
#128252=CARTESIAN_POINT('',(21.6997273401087,4.59542800405243,0.));
#128253=CARTESIAN_POINT('Origin',(20.9995498989716,4.96771895334164,0.));
#128254=CARTESIAN_POINT('',(20.9995498989716,4.96771895334164,0.));
#128255=CARTESIAN_POINT('',(21.6997273401087,4.59542800405243,0.));
#128256=CARTESIAN_POINT('',(20.9995498989716,4.96771895334164,400.));
#128257=CARTESIAN_POINT('',(21.6997273401087,4.59542800405243,400.));
#128258=CARTESIAN_POINT('',(20.9995498989716,4.96771895334164,0.));
#128259=CARTESIAN_POINT('Origin',(20.9995498989716,6.58171895334164,0.));
#128260=CARTESIAN_POINT('',(20.9995498989716,6.58171895334164,0.));
#128261=CARTESIAN_POINT('',(20.9995498989716,4.96771895334164,0.));
#128262=CARTESIAN_POINT('',(20.9995498989716,6.58171895334164,400.));
#128263=CARTESIAN_POINT('',(20.9995498989716,4.96771895334164,400.));
#128264=CARTESIAN_POINT('',(20.9995498989716,6.58171895334164,0.));
#128265=CARTESIAN_POINT('Origin',(19.9995498989716,6.58171895334164,0.));
#128266=CARTESIAN_POINT('',(19.2924368841731,7.28881950086129,0.));
#128267=CARTESIAN_POINT('Origin',(19.9995498989716,6.58171895334164,0.));
#128268=CARTESIAN_POINT('',(19.2924368841731,7.28881950086129,400.));
#128269=CARTESIAN_POINT('Origin',(19.9995498989716,6.58171895334164,400.));
#128270=CARTESIAN_POINT('',(19.2924368841731,7.28881950086129,0.));
#128271=CARTESIAN_POINT('Origin',(17.9142979170573,5.91065623501905,0.));
#128272=CARTESIAN_POINT('',(17.9142979170573,5.91065623501905,0.));
#128273=CARTESIAN_POINT('',(19.2924368841731,7.28881950086129,0.));
#128274=CARTESIAN_POINT('',(17.9142979170573,5.91065623501905,400.));
#128275=CARTESIAN_POINT('',(19.2924368841731,7.28881950086129,400.));
#128276=CARTESIAN_POINT('',(17.9142979170573,5.91065623501905,0.));
#128277=CARTESIAN_POINT('Origin',(21.4498629910497,2.37515349742076,0.));
#128278=CARTESIAN_POINT('',(16.449862991244,2.37510941893376,0.));
#128279=CARTESIAN_POINT('Origin',(21.4498629910497,2.37515349742076,0.));
#128280=CARTESIAN_POINT('',(16.449862991244,2.37510941893376,400.));
#128281=CARTESIAN_POINT('Origin',(21.4498629910497,2.37515349742076,400.));
#128282=CARTESIAN_POINT('',(16.449862991244,2.37510941893376,0.));
#128283=CARTESIAN_POINT('Origin',(16.4498705551123,1.5171094189671,0.));
#128284=CARTESIAN_POINT('',(16.4498705551123,1.5171094189671,0.));
#128285=CARTESIAN_POINT('',(16.449862991244,2.37510941893376,0.));
#128286=CARTESIAN_POINT('',(16.4498705551124,1.5171094189671,400.));
#128287=CARTESIAN_POINT('',(16.449862991244,2.37510941893376,400.));
#128288=CARTESIAN_POINT('',(16.4498705551123,1.5171094189671,0.));
#128289=CARTESIAN_POINT('Origin',(21.4498705549181,1.5171534974541,0.));
#128290=CARTESIAN_POINT('',(17.9143678173198,-2.01841157653832,0.));
#128291=CARTESIAN_POINT('Origin',(21.4498705549181,1.5171534974541,0.));
#128292=CARTESIAN_POINT('',(17.9143678173198,-2.01841157653832,400.));
#128293=CARTESIAN_POINT('Origin',(21.4498705549181,1.5171534974541,400.));
#128294=CARTESIAN_POINT('',(17.9143678173198,-2.01841157653832,0.));
#128295=CARTESIAN_POINT('Origin',(19.292531083162,-3.39655054365413,0.));
#128296=CARTESIAN_POINT('',(19.292531083162,-3.39655054365413,0.));
#128297=CARTESIAN_POINT('',(19.292531083162,-3.39655054365413,0.));
#128298=CARTESIAN_POINT('',(19.292531083162,-3.39655054365413,400.));
#128299=CARTESIAN_POINT('',(19.292531083162,-3.39655054365413,400.));
#128300=CARTESIAN_POINT('',(19.292531083162,-3.39655054365413,0.));
#128301=CARTESIAN_POINT('Origin',(19.9996316306817,-2.68943752885565,0.));
#128302=CARTESIAN_POINT('',(20.9996316305262,-2.68941989746085,0.));
#128303=CARTESIAN_POINT('Origin',(19.9996316306817,-2.68943752885565,0.));
#128304=CARTESIAN_POINT('',(20.9996316305262,-2.68941989746085,400.));
#128305=CARTESIAN_POINT('Origin',(19.9996316306817,-2.68943752885565,400.));
#128306=CARTESIAN_POINT('',(20.9996316305262,-2.68941989746085,0.));
#128307=CARTESIAN_POINT('Origin',(20.999603173455,-1.07541989771172,0.));
#128308=CARTESIAN_POINT('',(20.999603173455,-1.07541989771172,0.));
#128309=CARTESIAN_POINT('',(20.999603173455,-1.07541989771172,0.));
#128310=CARTESIAN_POINT('',(20.999603173455,-1.07541989771172,400.));
#128311=CARTESIAN_POINT('',(20.999603173455,-1.07541989771172,400.));
#128312=CARTESIAN_POINT('',(20.999603173455,-1.07541989771172,0.));
#128313=CARTESIAN_POINT('Origin',(21.6997740504746,-0.703116603375476,0.));
#128314=CARTESIAN_POINT('',(21.6997740504746,-0.703116603375476,0.));
#128315=CARTESIAN_POINT('',(21.6997740504746,-0.703116603375476,0.));
#128316=CARTESIAN_POINT('',(21.6997740504746,-0.703116603375476,400.));
#128317=CARTESIAN_POINT('',(21.6997740504746,-0.703116603375476,400.));
#128318=CARTESIAN_POINT('',(21.6997740504746,-0.703116603375476,0.));
#128319=CARTESIAN_POINT('Origin',(22.6997740503192,-0.703098971980677,0.));
#128320=CARTESIAN_POINT('',(22.6997740503192,-0.703098971980672,0.));
#128321=CARTESIAN_POINT('',(22.6997740503192,-0.703098971980677,0.));
#128322=CARTESIAN_POINT('',(22.6997740503192,-0.703098971980672,400.));
#128323=CARTESIAN_POINT('',(22.6997740503192,-0.703098971980677,400.));
#128324=CARTESIAN_POINT('',(22.6997740503192,-0.703098971980672,0.));
#128325=CARTESIAN_POINT('Origin',(22.6997793397376,-1.00309897193405,0.));
#128326=CARTESIAN_POINT('',(22.999779339691,-1.00309368251561,0.));
#128327=CARTESIAN_POINT('Origin',(22.6997793397376,-1.00309897193405,0.));
#128328=CARTESIAN_POINT('',(22.999779339691,-1.00309368251561,400.));
#128329=CARTESIAN_POINT('Origin',(22.6997793397376,-1.00309897193405,400.));
#128330=CARTESIAN_POINT('',(22.999779339691,-1.00309368251561,0.));
#128331=CARTESIAN_POINT('Origin',(22.9998507468399,-5.0530936818861,0.));
#128332=CARTESIAN_POINT('',(22.9998507468399,-5.0530936818861,0.));
#128333=CARTESIAN_POINT('',(22.9998507468399,-5.0530936818861,0.));
#128334=CARTESIAN_POINT('',(22.9998507468399,-5.0530936818861,400.));
#128335=CARTESIAN_POINT('',(22.9998507468399,-5.0530936818861,400.));
#128336=CARTESIAN_POINT('',(22.9998507468399,-5.0530936818861,0.));
#128337=CARTESIAN_POINT('Origin',(22.4998507469176,-5.0531024975835,0.));
#128338=CARTESIAN_POINT('',(22.499859562615,-5.55310249750579,0.));
#128339=CARTESIAN_POINT('Origin',(22.4998507469176,-5.0531024975835,0.));
#128340=CARTESIAN_POINT('',(22.499859562615,-5.55310249750579,400.));
#128341=CARTESIAN_POINT('Origin',(22.4998507469176,-5.0531024975835,400.));
#128342=CARTESIAN_POINT('',(22.499859562615,-5.55310249750579,0.));
#128343=CARTESIAN_POINT('Origin',(22.1638595626673,-5.55310842165444,0.));
#128344=CARTESIAN_POINT('',(22.1638595626673,-5.55310842165444,0.));
#128345=CARTESIAN_POINT('',(22.1638595626673,-5.55310842165444,0.));
#128346=CARTESIAN_POINT('',(22.1638595626673,-5.55310842165444,400.));
#128347=CARTESIAN_POINT('',(22.1638595626673,-5.55310842165444,400.));
#128348=CARTESIAN_POINT('',(22.1638595626673,-5.55310842165444,0.));
#128349=CARTESIAN_POINT('Origin',(22.1638771940621,-6.55310842149901,0.));
#128350=CARTESIAN_POINT('',(21.4567579457066,-5.84601410770119,0.));
#128351=CARTESIAN_POINT('Origin',(22.1638771940621,-6.55310842149901,0.));
#128352=CARTESIAN_POINT('',(21.4567579457066,-5.84601410770119,400.));
#128353=CARTESIAN_POINT('Origin',(22.1638771940621,-6.55310842149901,400.));
#128354=CARTESIAN_POINT('',(21.4567579457066,-5.84601410770119,0.));
#128355=CARTESIAN_POINT('Origin',(18.4996895254041,-8.80318680432375,0.));
#128356=CARTESIAN_POINT('',(18.4996895254041,-8.80318680432375,0.));
#128357=CARTESIAN_POINT('',(18.4996895254041,-8.80318680432375,0.));
#128358=CARTESIAN_POINT('',(18.4996895254041,-8.80318680432375,400.));
#128359=CARTESIAN_POINT('',(18.4996895254041,-8.80318680432375,400.));
#128360=CARTESIAN_POINT('',(18.4996895254041,-8.80318680432375,0.));
#128361=CARTESIAN_POINT('Origin',(18.4997027489502,-9.55318680420717,0.));
#128362=CARTESIAN_POINT('',(18.4997027489502,-9.55318680420717,0.));
#128363=CARTESIAN_POINT('',(18.4997027489502,-9.55318680420717,0.));
#128364=CARTESIAN_POINT('',(18.4997027489502,-9.55318680420717,400.));
#128365=CARTESIAN_POINT('',(18.4997027489502,-9.55318680420717,400.));
#128366=CARTESIAN_POINT('',(18.4997027489502,-9.55318680420717,0.));
#128367=CARTESIAN_POINT('Origin',(15.6380920610105,-12.4148984023017,0.));
#128368=CARTESIAN_POINT('',(15.6380920610105,-12.4148984023017,0.));
#128369=CARTESIAN_POINT('',(18.4997027489502,-9.55318680420717,0.));
#128370=CARTESIAN_POINT('',(15.6380920610105,-12.4148984023017,400.));
#128371=CARTESIAN_POINT('',(18.4997027489502,-9.55318680420717,400.));
#128372=CARTESIAN_POINT('',(15.6380920610105,-12.4148984023017,0.));
#128373=CARTESIAN_POINT('Origin',(15.4259562865038,-12.2027701081624,0.));
#128374=CARTESIAN_POINT('',(15.2545493290212,-12.4489806987683,0.));
#128375=CARTESIAN_POINT('Origin',(15.4259562865038,-12.2027701081624,0.));
#128376=CARTESIAN_POINT('',(15.2545493290212,-12.4489806987683,400.));
#128377=CARTESIAN_POINT('Origin',(15.4259562865038,-12.2027701081624,400.));
#128378=CARTESIAN_POINT('',(15.2545493290212,-12.4489806987683,0.));
#128379=CARTESIAN_POINT('Origin',(14.8102803067574,-13.0532372410527,0.));
#128380=CARTESIAN_POINT('',(15.250070467987,-13.6607609689548,0.));
#128381=CARTESIAN_POINT('Origin',(14.8102803067574,-13.0532372410527,0.));
#128382=CARTESIAN_POINT('',(15.250070467987,-13.6607609689548,400.));
#128383=CARTESIAN_POINT('Origin',(14.8102803067574,-13.0532372410527,400.));
#128384=CARTESIAN_POINT('',(15.2500702858638,-13.6607607173708,0.));
#128385=CARTESIAN_POINT('Origin',(15.4259862775064,-13.903770107898,0.));
#128386=CARTESIAN_POINT('',(15.6381145716457,-13.6916343333914,0.));
#128387=CARTESIAN_POINT('Origin',(15.4259862775064,-13.903770107898,0.));
#128388=CARTESIAN_POINT('',(15.6381145716457,-13.6916343333914,400.));
#128389=CARTESIAN_POINT('Origin',(15.4259862775064,-13.903770107898,400.));
#128390=CARTESIAN_POINT('',(15.6381145716457,-13.6916343333914,0.));
#128391=CARTESIAN_POINT('Origin',(18.4998261697403,-16.5532450213311,0.));
#128392=CARTESIAN_POINT('',(18.4998261697403,-16.5532450213311,0.));
#128393=CARTESIAN_POINT('',(18.4998261697403,-16.5532450213311,0.));
#128394=CARTESIAN_POINT('',(18.4998261697403,-16.5532450213311,400.));
#128395=CARTESIAN_POINT('',(18.4998261697403,-16.5532450213311,400.));
#128396=CARTESIAN_POINT('',(18.4998261697403,-16.5532450213311,0.));
#128397=CARTESIAN_POINT('Origin',(18.4998349854377,-17.0532450212534,0.));
#128398=CARTESIAN_POINT('',(18.4998349854377,-17.0532450212534,0.));
#128399=CARTESIAN_POINT('',(18.4998349854377,-17.0532450212534,400.));
#128400=CARTESIAN_POINT('Origin',(0.,1.9455,400.));
#128401=CARTESIAN_POINT('Origin',(0.,1.9455,0.));
#215596=UNCERTAINTY_MEASURE_WITH_UNIT(LENGTH_MEASURE(0.01),#215610,
'DISTANCE_ACCURACY_VALUE',
'Maximum model space distance between geometric entities at asserted c
onnectivities');
#215598=UNCERTAINTY_MEASURE_WITH_UNIT(LENGTH_MEASURE(0.01),#215610,
'DISTANCE_ACCURACY_VALUE',
'Maximum model space distance between geometric entities at asserted c
onnectivities');
#215607=(
GEOMETRIC_REPRESENTATION_CONTEXT(3)
GLOBAL_UNCERTAINTY_ASSIGNED_CONTEXT((#215596))
GLOBAL_UNIT_ASSIGNED_CONTEXT((#215610,#215612,#215613))
REPRESENTATION_CONTEXT('','3D')
);
#215609=(
GEOMETRIC_REPRESENTATION_CONTEXT(3)
GLOBAL_UNCERTAINTY_ASSIGNED_CONTEXT((#215598))
GLOBAL_UNIT_ASSIGNED_CONTEXT((#215610,#215612,#215613))
REPRESENTATION_CONTEXT('','3D')
);
#215610=(
LENGTH_UNIT()
NAMED_UNIT(*)
SI_UNIT(.MILLI.,.METRE.)
);
#215612=(
NAMED_UNIT(*)
PLANE_ANGLE_UNIT()
SI_UNIT($,.RADIAN.)
);
#215613=(
NAMED_UNIT(*)
SI_UNIT($,.STERADIAN.)
SOLID_ANGLE_UNIT()
);
#215622=SHAPE_DEFINITION_REPRESENTATION(#215634,#215651);
#215634=PRODUCT_DEFINITION_SHAPE('',$,#215662);
#215651=SHAPE_REPRESENTATION('',(#29550),#215607);
#215653=PRODUCT_DEFINITION_CONTEXT('part definition',#215685,'design');
#215662=PRODUCT_DEFINITION('2026-10-04-08-25-38-216','Barrel',#215672,#215653);
#215672=PRODUCT_DEFINITION_FORMATION('',$,#215695);
#215685=APPLICATION_CONTEXT(
'Core Data for Automotive Mechanical Design Process');
#215686=PRODUCT_CONTEXT('part definition',#215685,'mechanical');
#215695=PRODUCT('2026-10-04-08-25-38-216','Barrel',$,(#215686));
#215698=PRESENTATION_STYLE_ASSIGNMENT((#215700));
#215700=SURFACE_STYLE_USAGE(.BOTH.,#215702);
#215702=SURFACE_SIDE_STYLE('',(#215704));
#215704=SURFACE_STYLE_FILL_AREA(#215706);
#215706=FILL_AREA_STYLE('Opaque(245,245,246)',(#215708));
#215708=FILL_AREA_STYLE_COLOUR('Opaque(245,245,246)',#215710);
#215710=COLOUR_RGB('Opaque(245,245,246)', 0.66274510, 0.83137255, 0.94901961);
ENDSEC;
END-ISO-10303-21;
